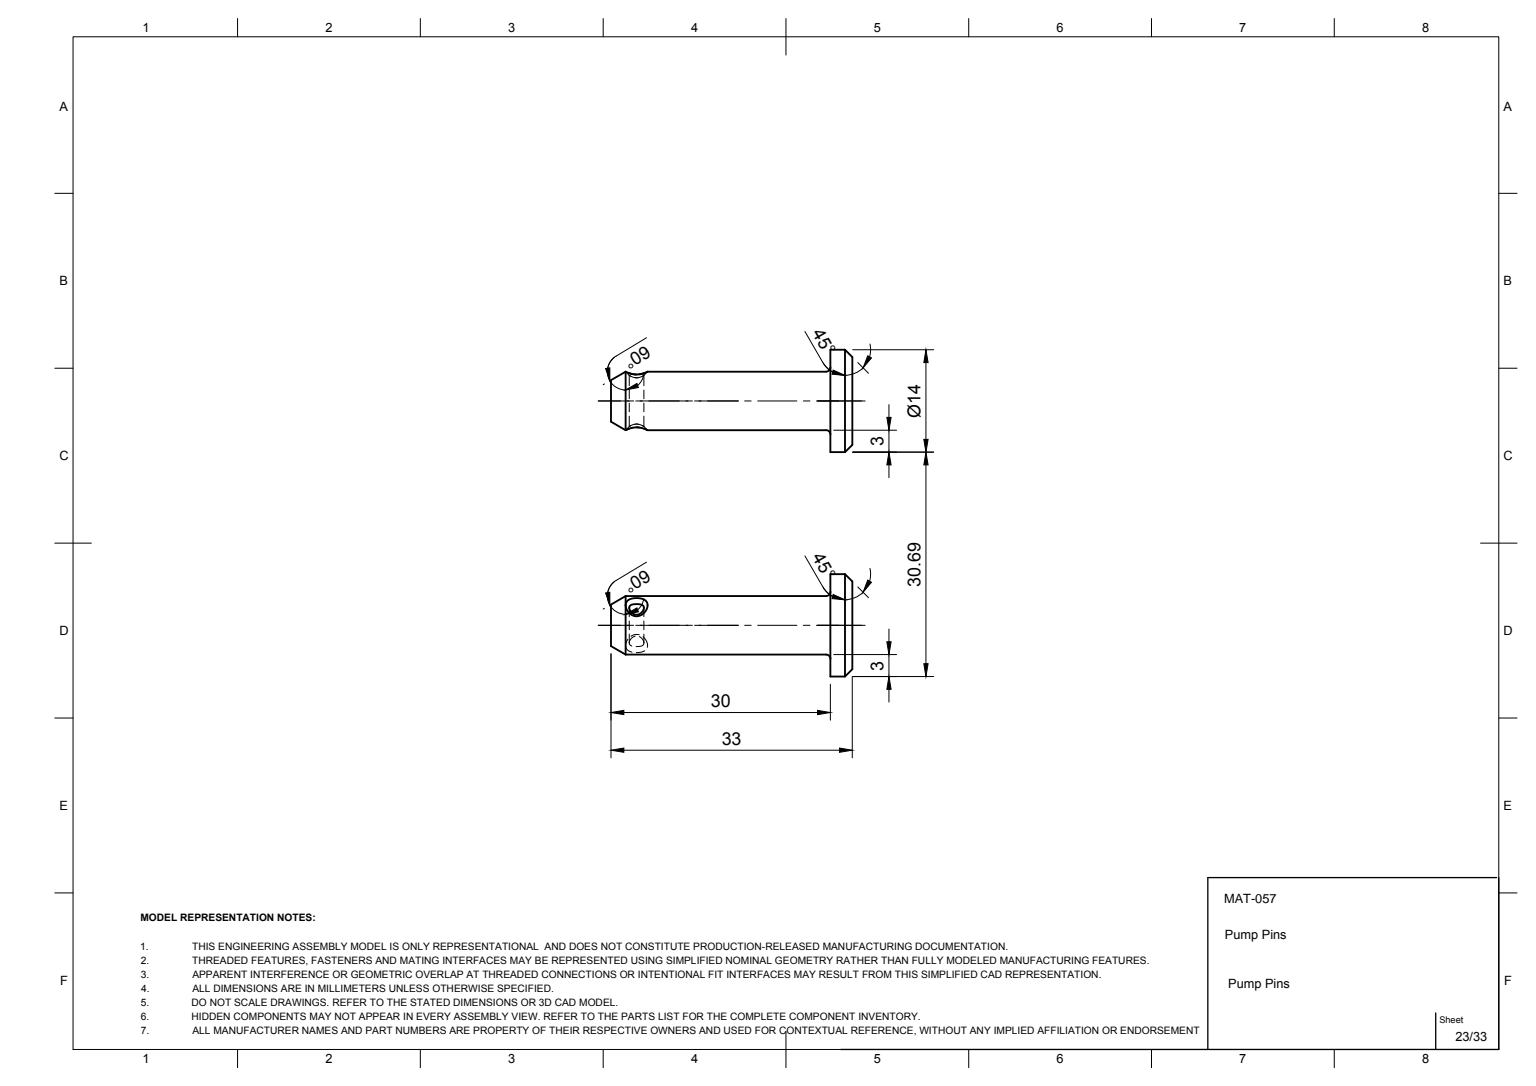
ISO-10303-21;
HEADER;
/* Generated by software containing ST-Developer
 * from STEP Tools, Inc. (www.steptools.com) 
 */

FILE_DESCRIPTION(
/* description */ ('STEP AP214', 'CAx-IF Rec.Pracs.---Representation and Presentation of Product Manufa
cturing Information (PMI)---4.0---2014-10-13'),
/* implementation_level */ '2;1');

FILE_NAME(
/* name */ 'Pump Pins.step',
/* time_stamp */ '2026-10-28T23:34:22+01:00',
/* author */ (''),
/* organization */ (''),
/* preprocessor_version */ 'ST-DEVELOPER v20.2',
/* originating_system */ 'Autodesk Translation Framework v15.17.0.0',
/* authorisation */ '');

FILE_SCHEMA (('AP242_MANAGED_MODEL_BASED_3D_ENGINEERING_MIM_LF { 1 0 10303 442 2 1 4 }'));
ENDSEC;

DATA;
#10=MECHANICAL_DESIGN_GEOMETRIC_PRESENTATION_REPRESENTATION('',(#264,#265),#27807);
#11=B_SPLINE_SURFACE_WITH_KNOTS('',1,3,((#21472,#21473,#21474,#21475,#21476,
#21477,#21478,#21479,#21480,#21481,#21482,#21483,#21484,#21485,#21486,#21487,
#21488,#21489),(#21490,#21491,#21492,#21493,#21494,#21495,#21496,#21497,
#21498,#21499,#21500,#21501,#21502,#21503,#21504,#21505,#21506,#21507)),
 .UNSPECIFIED.,.F.,.T.,.F.,(2,2),(4,2,2,2,2,2,2,2,4),(-5.33401314790998E-5,
1.0071581353373),(-0.00941606787651008,-0.00822939788115615,-0.00704272788580222,
-0.00585605789044829,-0.00466938789509436,-0.00348271789974043,-0.0022960479043865,
-0.00110937790903257,7.72920863213594E-5),.UNSPECIFIED.);
#12=B_SPLINE_SURFACE_WITH_KNOTS('',1,3,((#21574,#21575,#21576,#21577,#21578,
#21579,#21580,#21581,#21582,#21583,#21584,#21585,#21586,#21587,#21588,#21589,
#21590,#21591),(#21592,#21593,#21594,#21595,#21596,#21597,#21598,#21599,
#21600,#21601,#21602,#21603,#21604,#21605,#21606,#21607,#21608,#21609)),
 .UNSPECIFIED.,.F.,.T.,.F.,(2,2),(4,2,2,2,2,2,2,2,4),(-5.33401315292344E-5,
1.00729193620298),(-0.00941606787651008,-0.00822939788115615,-0.00704272788580222,
-0.00585605789044829,-0.00466938789509436,-0.00348271789974043,-0.0022960479043865,
-0.00110937790903257,7.72920863213577E-5),.UNSPECIFIED.);
#13=B_SPLINE_SURFACE_WITH_KNOTS('',1,3,((#21829,#21830,#21831,#21832,#21833,
#21834,#21835,#21836,#21837,#21838,#21839,#21840,#21841,#21842,#21843,#21844,
#21845,#21846),(#21847,#21848,#21849,#21850,#21851,#21852,#21853,#21854,
#21855,#21856,#21857,#21858,#21859,#21860,#21861,#21862,#21863,#21864)),
 .UNSPECIFIED.,.F.,.T.,.F.,(2,2),(4,2,2,2,2,2,2,2,4),(-4.93053323705934E-5,
1.01004399172031),(-0.00941606787651008,-0.00822939788115615,-0.00704272788580222,
-0.00585605789044829,-0.00466938789509436,-0.00348271789974043,-0.0022960479043865,
-0.00110937790903257,7.72920863213577E-5),.UNSPECIFIED.);
#14=B_SPLINE_SURFACE_WITH_KNOTS('',1,3,((#21865,#21866,#21867,#21868,#21869,
#21870,#21871,#21872,#21873,#21874,#21875,#21876,#21877,#21878,#21879,#21880,
#21881,#21882),(#21883,#21884,#21885,#21886,#21887,#21888,#21889,#21890,
#21891,#21892,#21893,#21894,#21895,#21896,#21897,#21898,#21899,#21900)),
 .UNSPECIFIED.,.F.,.T.,.F.,(2,2),(4,2,2,2,2,2,2,2,4),(-4.93053323625481E-5,
1.01010892051971),(-0.00941606787651008,-0.00822939788115615,-0.00704272788580222,
-0.00585605789044829,-0.00466938789509436,-0.00348271789974043,-0.0022960479043865,
-0.00110937790903257,7.72920863213594E-5),.UNSPECIFIED.);
#15=B_SPLINE_SURFACE_WITH_KNOTS('',1,3,((#21901,#21902,#21903,#21904,#21905,
#21906,#21907,#21908,#21909,#21910,#21911,#21912,#21913,#21914,#21915,#21916,
#21917,#21918),(#21919,#21920,#21921,#21922,#21923,#21924,#21925,#21926,
#21927,#21928,#21929,#21930,#21931,#21932,#21933,#21934,#21935,#21936)),
 .UNSPECIFIED.,.F.,.T.,.F.,(2,2),(4,2,2,2,2,2,2,2,4),(-4.62400267622051E-5,
1.00715813533735),(-0.00941606787651008,-0.00822939788115615,-0.00704272788580222,
-0.00585605789044829,-0.00466938789509436,-0.00348271789974043,-0.0022960479043865,
-0.00110937790903257,7.72920863213594E-5),.UNSPECIFIED.);
#16=B_SPLINE_SURFACE_WITH_KNOTS('',1,3,((#22003,#22004,#22005,#22006,#22007,
#22008,#22009,#22010,#22011,#22012,#22013,#22014,#22015,#22016,#22017,#22018,
#22019,#22020),(#22021,#22022,#22023,#22024,#22025,#22026,#22027,#22028,
#22029,#22030,#22031,#22032,#22033,#22034,#22035,#22036,#22037,#22038)),
 .UNSPECIFIED.,.F.,.T.,.F.,(2,2),(4,2,2,2,2,2,2,2,4),(-4.62400267636951E-5,
1.00729193620287),(-0.00941606787651008,-0.00822939788115615,-0.00704272788580222,
-0.00585605789044829,-0.00466938789509436,-0.00348271789974043,-0.0022960479043865,
-0.00110937790903257,7.72920863213577E-5),.UNSPECIFIED.);
#17=B_SPLINE_SURFACE_WITH_KNOTS('',1,3,((#22258,#22259,#22260,#22261,#22262,
#22263,#22264,#22265,#22266,#22267,#22268,#22269,#22270,#22271,#22272,#22273,
#22274,#22275),(#22276,#22277,#22278,#22279,#22280,#22281,#22282,#22283,
#22284,#22285,#22286,#22287,#22288,#22289,#22290,#22291,#22292,#22293)),
 .UNSPECIFIED.,.F.,.T.,.F.,(2,2),(4,2,2,2,2,2,2,2,4),(-4.93053323759633E-5,
1.00770004007163),(-0.00941606787651008,-0.00822939788115615,-0.00704272788580222,
-0.00585605789044829,-0.00466938789509436,-0.00348271789974043,-0.0022960479043865,
-0.00110937790903257,7.72920863213577E-5),.UNSPECIFIED.);
#18=B_SPLINE_SURFACE_WITH_KNOTS('',1,3,((#22294,#22295,#22296,#22297,#22298,
#22299,#22300,#22301,#22302,#22303,#22304,#22305,#22306,#22307,#22308,#22309,
#22310,#22311),(#22312,#22313,#22314,#22315,#22316,#22317,#22318,#22319,
#22320,#22321,#22322,#22323,#22324,#22325,#22326,#22327,#22328,#22329)),
 .UNSPECIFIED.,.F.,.T.,.F.,(2,2),(4,2,2,2,2,2,2,2,4),(-4.93053323767007E-5,
1.00811188664),(-0.00941606787651008,-0.00822939788115615,-0.00704272788580222,
-0.00585605789044829,-0.00466938789509436,-0.00348271789974043,-0.0022960479043865,
-0.00110937790903257,7.72920863213594E-5),.UNSPECIFIED.);
#218=SHAPE_REPRESENTATION_RELATIONSHIP('SRR','None',#27915,#240);
#240=ADVANCED_BREP_SHAPE_REPRESENTATION('',(#293,#294),#27795);
#264=STYLED_ITEM('',(#28063),#293);
#265=STYLED_ITEM('',(#28063),#294);
#293=MANIFOLD_SOLID_BREP('Body1',#12040);
#294=MANIFOLD_SOLID_BREP('Body2',#12041);
#414=FACE_BOUND('',#2492,.T.);
#415=FACE_BOUND('',#2506,.T.);
#665=PLANE('',#13280);
#666=PLANE('',#13281);
#667=PLANE('',#13282);
#668=PLANE('',#13299);
#669=PLANE('',#13300);
#670=PLANE('',#13301);
#832=TOROIDAL_SURFACE('',#13271,4.59999999999999,0.6);
#833=TOROIDAL_SURFACE('',#13290,4.59999999999999,0.6);
#904=B_SPLINE_CURVE_WITH_KNOTS('',3,(#21510,#21511,#21512,#21513,#21514,
#21515,#21516,#21517,#21518,#21519,#21520,#21521,#21522,#21523,#21524,#21525,
#21526,#21527,#21528,#21529,#21530,#21531,#21532,#21533,#21534,#21535,#21536,
#21537,#21538,#21539,#21540,#21541,#21542,#21543,#21544,#21545,#21546,#21547),
 .UNSPECIFIED.,.F.,.F.,(4,2,2,2,2,2,2,2,2,2,2,2,2,2,2,2,2,2,4),(1.00089634517109E-6,
0.0135124805886909,0.0270102893796787,0.0542554527433717,0.0725924484028551,
0.0831509031929542,0.0939203394783847,0.114150905777324,0.132564433691206,
0.163148633358063,0.193616759129243,0.211927287774423,0.23206669119174,
0.242799260198686,0.253302631405238,0.27156325585088,0.298722401714205,
0.312167688321445,0.325612440221502),.UNSPECIFIED.);
#905=B_SPLINE_CURVE_WITH_KNOTS('',3,(#21551,#21552,#21553,#21554,#21555,
#21556,#21557,#21558,#21559,#21560,#21561,#21562,#21563,#21564,#21565,#21566,
#21567,#21568,#21569,#21570,#21571,#21572),.UNSPECIFIED.,.F.,.F.,(4,2,2,
2,2,2,2,2,2,2,4),(0.,0.0625283246425461,0.0937924869638204,0.125056649285095,
0.187584973927639,0.250113298570183,0.312641623212727,0.343905785533998,
0.359537866694632,0.375169947855267,0.500226597140354),.UNSPECIFIED.);
#906=B_SPLINE_CURVE_WITH_KNOTS('',3,(#21612,#21613,#21614,#21615,#21616,
#21617,#21618,#21619,#21620,#21621,#21622,#21623,#21624,#21625,#21626,#21627,
#21628,#21629,#21630,#21631,#21632,#21633,#21634,#21635,#21636,#21637,#21638,
#21639,#21640,#21641,#21642,#21643,#21644,#21645,#21646,#21647,#21648,#21649),
 .UNSPECIFIED.,.F.,.F.,(4,2,2,2,2,2,2,2,2,2,2,2,2,2,2,2,2,2,4),(1.00089547843557E-6,
0.0135124805885893,0.0270102893791961,0.0542554527419749,0.072592448400889,
0.0831509031907464,0.0939203394761004,0.1141509057748,0.132564433688463,
0.163148633354892,0.193616759125631,0.211927287770558,0.232066691187639,
0.242799260194547,0.253302631400942,0.271563255846155,0.298722401708962,
0.312167688315685,0.325612440214992),.UNSPECIFIED.);
#907=B_SPLINE_CURVE_WITH_KNOTS('',3,(#21653,#21654,#21655,#21656,#21657,
#21658,#21659,#21660,#21661,#21662,#21663,#21664,#21665,#21666,#21667,#21668,
#21669,#21670,#21671,#21672,#21673,#21674),.UNSPECIFIED.,.F.,.F.,(4,2,2,
2,2,2,2,2,2,2,4),(0.,0.0625305420531017,0.0937958130796483,0.125061084106195,
0.187591626159283,0.250122168212371,0.31265271026546,0.343917981292008,
0.359550616805279,0.37518325231855,0.500244336424745),.UNSPECIFIED.);
#908=B_SPLINE_CURVE_WITH_KNOTS('',3,(#21677,#21678,#21679,#21680,#21681,
#21682,#21683,#21684,#21685,#21686,#21687,#21688,#21689,#21690,#21691,#21692,
#21693,#21694,#21695,#21696,#21697,#21698,#21699,#21700,#21701,#21702,#21703,
#21704,#21705,#21706,#21707,#21708,#21709,#21710,#21711,#21712,#21713,#21714),
 .UNSPECIFIED.,.F.,.F.,(4,2,2,2,2,2,2,2,2,2,2,2,2,2,2,2,2,2,4),(0.,0.0303468331885949,
0.0404805816100016,0.0838349998679533,0.0899468517242951,0.0960856059764287,
0.119205002215768,0.140283020185445,0.159234503235151,0.176557837747224,
0.209013384982688,0.227277173706207,0.247357834439419,0.25806173913776,
0.268531153677092,0.286711917123732,0.300273063907743,0.310385248581606,
0.340667271090375),.UNSPECIFIED.);
#909=B_SPLINE_CURVE_WITH_KNOTS('',3,(#21716,#21717,#21718,#21719,#21720,
#21721,#21722,#21723,#21724,#21725,#21726,#21727,#21728,#21729,#21730,#21731,
#21732,#21733,#21734,#21735,#21736,#21737,#21738,#21739,#21740,#21741,#21742,
#21743,#21744,#21745,#21746,#21747,#21748,#21749,#21750,#21751,#21752,#21753),
 .UNSPECIFIED.,.F.,.F.,(4,2,2,2,2,2,2,2,2,2,2,2,2,2,2,2,2,2,4),(0.,0.0303468331885437,
0.0404805816098057,0.0838349998664512,0.0899468517228076,0.096085605973945,
0.119205002207746,0.140283020172398,0.159234503217531,0.176557837725533,
0.209013384952252,0.227277173670161,0.247357834397049,0.258061739092016,
0.268531153628422,0.286711917069987,0.300273063850531,0.310385248521581,
0.340667271021422),.UNSPECIFIED.);
#910=B_SPLINE_CURVE_WITH_KNOTS('',3,(#21764,#21765,#21766,#21767,#21768,
#21769,#21770,#21771,#21772,#21773,#21774,#21775,#21776,#21777,#21778,#21779,
#21780,#21781,#21782,#21783,#21784,#21785),.UNSPECIFIED.,.F.,.F.,(4,2,2,
2,2,2,2,2,2,2,4),(0.500226597140354,0.562698272497809,0.593934110176538,
0.625169947855266,0.687641623212725,0.750113298570185,0.812584973927644,
0.843820811606377,0.859438730445742,0.875056649285107,1.),.UNSPECIFIED.);
#911=B_SPLINE_CURVE_WITH_KNOTS('',3,(#21786,#21787,#21788,#21789,#21790,
#21791,#21792,#21793,#21794,#21795,#21796,#21797,#21798,#21799,#21800,#21801,
#21802,#21803,#21804,#21805,#21806,#21807,#21808,#21809),.UNSPECIFIED.,
 .F.,.F.,(4,2,2,2,2,2,2,2,2,2,2,4),(0.500244336424745,0.56271379437167,
0.593948523345132,0.609565887831865,0.625183252318598,0.687652710265505,
0.750122168212412,0.812591626159318,0.843826355132767,0.859443719619489,
0.87506108410621,1.),.UNSPECIFIED.);
#912=B_SPLINE_CURVE_WITH_KNOTS('',3,(#21939,#21940,#21941,#21942,#21943,
#21944,#21945,#21946,#21947,#21948,#21949,#21950,#21951,#21952,#21953,#21954,
#21955,#21956,#21957,#21958,#21959,#21960,#21961,#21962,#21963,#21964,#21965,
#21966,#21967,#21968,#21969,#21970,#21971,#21972,#21973,#21974,#21975,#21976),
 .UNSPECIFIED.,.F.,.F.,(4,2,2,2,2,2,2,2,2,2,2,2,2,2,2,2,2,2,4),(1.00089633934029E-6,
0.0135124805888077,0.0270102893800241,0.0542554527437976,0.0725924484033422,
0.0831509031934888,0.0939203394789252,0.114150905777859,0.132564433691779,
0.163148633358663,0.193616759129903,0.211927287775115,0.232066691192426,
0.242799260199493,0.253302631405774,0.271563255850625,0.298722401712991,
0.312167688319558,0.32561244021873),.UNSPECIFIED.);
#913=B_SPLINE_CURVE_WITH_KNOTS('',3,(#21980,#21981,#21982,#21983,#21984,
#21985,#21986,#21987,#21988,#21989,#21990,#21991,#21992,#21993,#21994,#21995,
#21996,#21997,#21998,#21999,#22000,#22001),.UNSPECIFIED.,.F.,.F.,(4,2,2,
2,2,2,2,2,2,2,4),(0.,0.062528324642553,0.0937924869638229,0.125056649285093,
0.187584973927634,0.250113298570175,0.312641623212717,0.343905785533987,
0.359537866694625,0.375169947855263,0.500226597140362),.UNSPECIFIED.);
#914=B_SPLINE_CURVE_WITH_KNOTS('',3,(#22041,#22042,#22043,#22044,#22045,
#22046,#22047,#22048,#22049,#22050,#22051,#22052,#22053,#22054,#22055,#22056,
#22057,#22058,#22059,#22060,#22061,#22062,#22063,#22064,#22065,#22066,#22067,
#22068,#22069,#22070,#22071,#22072,#22073,#22074,#22075,#22076,#22077,#22078),
 .UNSPECIFIED.,.F.,.F.,(4,2,2,2,2,2,2,2,2,2,2,2,2,2,2,2,2,2,4),(1.00089547198642E-6,
0.0135124805886458,0.0270102893792894,0.0542554527414999,0.0725924484001046,
0.0831509031898948,0.0939203394752058,0.114150905773714,0.132564433687167,
0.163148633353336,0.193616759123885,0.211927287768641,0.232066691185389,
0.242799260192144,0.253302631398652,0.27156325584398,0.29872240170682,0.312167688313921,
0.32561244021362),.UNSPECIFIED.);
#915=B_SPLINE_CURVE_WITH_KNOTS('',3,(#22082,#22083,#22084,#22085,#22086,
#22087,#22088,#22089,#22090,#22091,#22092,#22093,#22094,#22095,#22096,#22097,
#22098,#22099,#22100,#22101,#22102,#22103),.UNSPECIFIED.,.F.,.F.,(4,2,2,
2,2,2,2,2,2,2,4),(0.,0.0625305420531068,0.0937958130796515,0.125061084106196,
0.187591626159282,0.250122168212368,0.312652710265454,0.343917981291998,
0.359550616805267,0.375183252318535,0.500244336424746),.UNSPECIFIED.);
#916=B_SPLINE_CURVE_WITH_KNOTS('',3,(#22106,#22107,#22108,#22109,#22110,
#22111,#22112,#22113,#22114,#22115,#22116,#22117,#22118,#22119,#22120,#22121,
#22122,#22123,#22124,#22125,#22126,#22127,#22128,#22129,#22130,#22131,#22132,
#22133,#22134,#22135,#22136,#22137,#22138,#22139,#22140,#22141,#22142,#22143),
 .UNSPECIFIED.,.F.,.F.,(4,2,2,2,2,2,2,2,2,2,2,2,2,2,2,2,2,2,4),(0.,0.0303468331886201,
0.0404805816100005,0.0838349998685196,0.0899468517249421,0.0960856059763945,
0.119205002212153,0.140283020178524,0.159234503225117,0.176557837734437,
0.209013384964693,0.227277173685149,0.247357834414858,0.25806173911128,
0.268531153648718,0.286711917091893,0.300273063873447,0.310385248545583,
0.340667271049151),.UNSPECIFIED.);
#917=B_SPLINE_CURVE_WITH_KNOTS('',3,(#22145,#22146,#22147,#22148,#22149,
#22150,#22151,#22152,#22153,#22154,#22155,#22156,#22157,#22158,#22159,#22160,
#22161,#22162,#22163,#22164,#22165,#22166,#22167,#22168,#22169,#22170,#22171,
#22172,#22173,#22174,#22175,#22176,#22177,#22178,#22179,#22180,#22181,#22182),
 .UNSPECIFIED.,.F.,.F.,(4,2,2,2,2,2,2,2,2,2,2,2,2,2,2,2,2,2,4),(0.,0.0303468331885424,
0.0404805816097377,0.0838349998665984,0.0899468517222195,0.0960856059733606,
0.119205002209305,0.140283020175775,0.159234503222523,0.176557837732021,
0.209013384962109,0.227277173682202,0.247357834411472,0.258061739107788,
0.268531153645427,0.28671191708922,0.300273063871285,0.310385248543308,
0.340667271045991),.UNSPECIFIED.);
#918=B_SPLINE_CURVE_WITH_KNOTS('',3,(#22193,#22194,#22195,#22196,#22197,
#22198,#22199,#22200,#22201,#22202,#22203,#22204,#22205,#22206,#22207,#22208,
#22209,#22210,#22211,#22212,#22213,#22214),.UNSPECIFIED.,.F.,.F.,(4,2,2,
2,2,2,2,2,2,2,4),(0.500226597140362,0.562698272497811,0.593934110176537,
0.625169947855262,0.687641623212722,0.750113298570183,0.812584973927644,
0.843820811606372,0.859438730445736,0.875056649285099,1.),.UNSPECIFIED.);
#919=B_SPLINE_CURVE_WITH_KNOTS('',3,(#22215,#22216,#22217,#22218,#22219,
#22220,#22221,#22222,#22223,#22224,#22225,#22226,#22227,#22228,#22229,#22230,
#22231,#22232,#22233,#22234,#22235,#22236,#22237,#22238),.UNSPECIFIED.,
 .F.,.F.,(4,2,2,2,2,2,2,2,2,2,2,4),(0.500244336424746,0.562713794371627,
0.593948523345067,0.609565887831793,0.625183252318519,0.687652710265425,
0.75012216821233,0.812591626159236,0.843826355132694,0.859443719619418,
0.875061084106143,1.),.UNSPECIFIED.);
#1151=CYLINDRICAL_SURFACE('',#13264,1.);
#1152=CYLINDRICAL_SURFACE('',#13269,4.);
#1153=CYLINDRICAL_SURFACE('',#13274,6.99999999999999);
#1154=CYLINDRICAL_SURFACE('',#13283,1.);
#1155=CYLINDRICAL_SURFACE('',#13288,4.00000000000001);
#1156=CYLINDRICAL_SURFACE('',#13293,7.);
#1706=FACE_OUTER_BOUND('',#2482,.T.);
#1707=FACE_OUTER_BOUND('',#2483,.T.);
#1708=FACE_OUTER_BOUND('',#2484,.T.);
#1709=FACE_OUTER_BOUND('',#2485,.T.);
#1710=FACE_OUTER_BOUND('',#2486,.T.);
#1711=FACE_OUTER_BOUND('',#2487,.T.);
#1712=FACE_OUTER_BOUND('',#2488,.T.);
#1713=FACE_OUTER_BOUND('',#2489,.T.);
#1714=FACE_OUTER_BOUND('',#2490,.T.);
#1715=FACE_OUTER_BOUND('',#2491,.T.);
#1716=FACE_OUTER_BOUND('',#2493,.T.);
#1717=FACE_OUTER_BOUND('',#2494,.T.);
#1718=FACE_OUTER_BOUND('',#2495,.T.);
#1719=FACE_OUTER_BOUND('',#2496,.T.);
#1720=FACE_OUTER_BOUND('',#2497,.T.);
#1721=FACE_OUTER_BOUND('',#2498,.T.);
#1722=FACE_OUTER_BOUND('',#2499,.T.);
#1723=FACE_OUTER_BOUND('',#2500,.T.);
#1724=FACE_OUTER_BOUND('',#2501,.T.);
#1725=FACE_OUTER_BOUND('',#2502,.T.);
#1726=FACE_OUTER_BOUND('',#2503,.T.);
#1727=FACE_OUTER_BOUND('',#2504,.T.);
#1728=FACE_OUTER_BOUND('',#2505,.T.);
#1729=FACE_OUTER_BOUND('',#2507,.T.);
#1730=FACE_OUTER_BOUND('',#2508,.T.);
#1731=FACE_OUTER_BOUND('',#2509,.T.);
#2482=EDGE_LOOP('',(#10163,#10164,#10165,#10166));
#2483=EDGE_LOOP('',(#10167,#10168,#10169,#10170));
#2484=EDGE_LOOP('',(#10171,#10172,#10173,#10174,#10175,#10176));
#2485=EDGE_LOOP('',(#10177,#10178,#10179,#10180,#10181));
#2486=EDGE_LOOP('',(#10182,#10183,#10184,#10185,#10186,#10187,#10188,#10189,
#10190));
#2487=EDGE_LOOP('',(#10191,#10192,#10193,#10194));
#2488=EDGE_LOOP('',(#10195,#10196,#10197,#10198,#10199));
#2489=EDGE_LOOP('',(#10200,#10201,#10202,#10203,#10204));
#2490=EDGE_LOOP('',(#10205));
#2491=EDGE_LOOP('',(#10206));
#2492=EDGE_LOOP('',(#10207));
#2493=EDGE_LOOP('',(#10208));
#2494=EDGE_LOOP('',(#10209,#10210,#10211,#10212));
#2495=EDGE_LOOP('',(#10213,#10214,#10215,#10216));
#2496=EDGE_LOOP('',(#10217,#10218,#10219,#10220));
#2497=EDGE_LOOP('',(#10221,#10222,#10223,#10224));
#2498=EDGE_LOOP('',(#10225,#10226,#10227,#10228,#10229,#10230));
#2499=EDGE_LOOP('',(#10231,#10232,#10233,#10234,#10235));
#2500=EDGE_LOOP('',(#10236,#10237,#10238,#10239,#10240,#10241,#10242,#10243,
#10244));
#2501=EDGE_LOOP('',(#10245,#10246,#10247,#10248));
#2502=EDGE_LOOP('',(#10249,#10250,#10251,#10252,#10253));
#2503=EDGE_LOOP('',(#10254,#10255,#10256,#10257,#10258));
#2504=EDGE_LOOP('',(#10259));
#2505=EDGE_LOOP('',(#10260));
#2506=EDGE_LOOP('',(#10261));
#2507=EDGE_LOOP('',(#10262));
#2508=EDGE_LOOP('',(#10263,#10264,#10265,#10266));
#2509=EDGE_LOOP('',(#10267,#10268,#10269,#10270));
#3344=LINE('',#21549,#4164);
#3345=LINE('',#21573,#4165);
#3346=LINE('',#21651,#4166);
#3347=LINE('',#21675,#4167);
#3348=LINE('',#21715,#4168);
#3349=LINE('',#21757,#4169);
#3350=LINE('',#21763,#4170);
#3351=LINE('',#21820,#4171);
#3352=LINE('',#21824,#4172);
#3353=LINE('',#21978,#4173);
#3354=LINE('',#22002,#4174);
#3355=LINE('',#22080,#4175);
#3356=LINE('',#22104,#4176);
#3357=LINE('',#22144,#4177);
#3358=LINE('',#22186,#4178);
#3359=LINE('',#22192,#4179);
#3360=LINE('',#22249,#4180);
#3361=LINE('',#22253,#4181);
#4164=VECTOR('',#16254,10.);
#4165=VECTOR('',#16255,10.);
#4166=VECTOR('',#16256,10.);
#4167=VECTOR('',#16257,10.);
#4168=VECTOR('',#16260,1.);
#4169=VECTOR('',#16265,4.);
#4170=VECTOR('',#16274,4.);
#4171=VECTOR('',#16287,6.99999999999999);
#4172=VECTOR('',#16292,5.99999999999997);
#4173=VECTOR('',#16301,10.);
#4174=VECTOR('',#16302,10.);
#4175=VECTOR('',#16303,10.);
#4176=VECTOR('',#16304,10.);
#4177=VECTOR('',#16307,1.);
#4178=VECTOR('',#16312,4.00000000000001);
#4179=VECTOR('',#16321,4.00000000000001);
#4180=VECTOR('',#16334,7.);
#4181=VECTOR('',#16339,5.99999999999998);
#4833=CIRCLE('',#13266,4.);
#4834=CIRCLE('',#13267,2.84529946162073);
#4835=CIRCLE('',#13268,4.);
#4836=CIRCLE('',#13270,4.);
#4837=CIRCLE('',#13272,4.59999999999999);
#4838=CIRCLE('',#13273,0.6);
#4839=CIRCLE('',#13275,6.99999999999999);
#4840=CIRCLE('',#13276,6.99999999999999);
#4841=CIRCLE('',#13277,6.99999999999999);
#4842=CIRCLE('',#13279,5.99999999999997);
#4843=CIRCLE('',#13285,4.00000000000001);
#4844=CIRCLE('',#13286,2.84529946162074);
#4845=CIRCLE('',#13287,4.00000000000001);
#4846=CIRCLE('',#13289,4.00000000000001);
#4847=CIRCLE('',#13291,4.6);
#4848=CIRCLE('',#13292,0.6);
#4849=CIRCLE('',#13294,7.);
#4850=CIRCLE('',#13295,7.);
#4851=CIRCLE('',#13296,7.);
#4852=CIRCLE('',#13298,5.99999999999998);
#5781=VERTEX_POINT('',#21508);
#5782=VERTEX_POINT('',#21509);
#5783=VERTEX_POINT('',#21548);
#5784=VERTEX_POINT('',#21550);
#5785=VERTEX_POINT('',#21610);
#5786=VERTEX_POINT('',#21611);
#5787=VERTEX_POINT('',#21650);
#5788=VERTEX_POINT('',#21652);
#5789=VERTEX_POINT('',#21756);
#5790=VERTEX_POINT('',#21761);
#5791=VERTEX_POINT('',#21811);
#5792=VERTEX_POINT('',#21815);
#5793=VERTEX_POINT('',#21816);
#5794=VERTEX_POINT('',#21819);
#5795=VERTEX_POINT('',#21823);
#5796=VERTEX_POINT('',#21937);
#5797=VERTEX_POINT('',#21938);
#5798=VERTEX_POINT('',#21977);
#5799=VERTEX_POINT('',#21979);
#5800=VERTEX_POINT('',#22039);
#5801=VERTEX_POINT('',#22040);
#5802=VERTEX_POINT('',#22079);
#5803=VERTEX_POINT('',#22081);
#5804=VERTEX_POINT('',#22185);
#5805=VERTEX_POINT('',#22190);
#5806=VERTEX_POINT('',#22240);
#5807=VERTEX_POINT('',#22244);
#5808=VERTEX_POINT('',#22245);
#5809=VERTEX_POINT('',#22248);
#5810=VERTEX_POINT('',#22252);
#7294=EDGE_CURVE('',#5781,#5782,#904,.T.);
#7295=EDGE_CURVE('',#5781,#5783,#3344,.T.);
#7296=EDGE_CURVE('',#5784,#5783,#905,.T.);
#7297=EDGE_CURVE('',#5782,#5784,#3345,.T.);
#7298=EDGE_CURVE('',#5785,#5786,#906,.T.);
#7299=EDGE_CURVE('',#5785,#5787,#3346,.T.);
#7300=EDGE_CURVE('',#5788,#5787,#907,.T.);
#7301=EDGE_CURVE('',#5786,#5788,#3347,.T.);
#7302=EDGE_CURVE('',#5782,#5781,#908,.T.);
#7303=EDGE_CURVE('',#5781,#5785,#3348,.T.);
#7304=EDGE_CURVE('',#5786,#5785,#909,.T.);
#7305=EDGE_CURVE('',#5784,#5788,#4833,.T.);
#7306=EDGE_CURVE('',#5784,#5789,#3349,.T.);
#7307=EDGE_CURVE('',#5789,#5789,#4834,.T.);
#7308=EDGE_CURVE('',#5788,#5784,#4835,.T.);
#7309=EDGE_CURVE('',#5790,#5790,#4836,.T.);
#7310=EDGE_CURVE('',#5790,#5783,#3350,.T.);
#7311=EDGE_CURVE('',#5783,#5784,#910,.T.);
#7312=EDGE_CURVE('',#5787,#5788,#911,.T.);
#7313=EDGE_CURVE('',#5791,#5791,#4837,.T.);
#7314=EDGE_CURVE('',#5791,#5790,#4838,.T.);
#7315=EDGE_CURVE('',#5792,#5793,#4839,.T.);
#7316=EDGE_CURVE('',#5793,#5792,#4840,.T.);
#7317=EDGE_CURVE('',#5793,#5794,#3351,.T.);
#7318=EDGE_CURVE('',#5794,#5794,#4841,.T.);
#7319=EDGE_CURVE('',#5792,#5795,#3352,.T.);
#7320=EDGE_CURVE('',#5795,#5795,#4842,.T.);
#7321=EDGE_CURVE('',#5796,#5797,#912,.T.);
#7322=EDGE_CURVE('',#5796,#5798,#3353,.T.);
#7323=EDGE_CURVE('',#5799,#5798,#913,.T.);
#7324=EDGE_CURVE('',#5797,#5799,#3354,.T.);
#7325=EDGE_CURVE('',#5800,#5801,#914,.T.);
#7326=EDGE_CURVE('',#5800,#5802,#3355,.T.);
#7327=EDGE_CURVE('',#5803,#5802,#915,.T.);
#7328=EDGE_CURVE('',#5801,#5803,#3356,.T.);
#7329=EDGE_CURVE('',#5797,#5796,#916,.T.);
#7330=EDGE_CURVE('',#5796,#5800,#3357,.T.);
#7331=EDGE_CURVE('',#5801,#5800,#917,.T.);
#7332=EDGE_CURVE('',#5799,#5803,#4843,.T.);
#7333=EDGE_CURVE('',#5799,#5804,#3358,.T.);
#7334=EDGE_CURVE('',#5804,#5804,#4844,.T.);
#7335=EDGE_CURVE('',#5803,#5799,#4845,.T.);
#7336=EDGE_CURVE('',#5805,#5805,#4846,.T.);
#7337=EDGE_CURVE('',#5805,#5798,#3359,.T.);
#7338=EDGE_CURVE('',#5798,#5799,#918,.T.);
#7339=EDGE_CURVE('',#5802,#5803,#919,.T.);
#7340=EDGE_CURVE('',#5806,#5806,#4847,.T.);
#7341=EDGE_CURVE('',#5806,#5805,#4848,.T.);
#7342=EDGE_CURVE('',#5807,#5808,#4849,.T.);
#7343=EDGE_CURVE('',#5808,#5807,#4850,.T.);
#7344=EDGE_CURVE('',#5808,#5809,#3360,.T.);
#7345=EDGE_CURVE('',#5809,#5809,#4851,.T.);
#7346=EDGE_CURVE('',#5807,#5810,#3361,.T.);
#7347=EDGE_CURVE('',#5810,#5810,#4852,.T.);
#10163=ORIENTED_EDGE('',*,*,#7294,.F.);
#10164=ORIENTED_EDGE('',*,*,#7295,.T.);
#10165=ORIENTED_EDGE('',*,*,#7296,.F.);
#10166=ORIENTED_EDGE('',*,*,#7297,.F.);
#10167=ORIENTED_EDGE('',*,*,#7298,.F.);
#10168=ORIENTED_EDGE('',*,*,#7299,.T.);
#10169=ORIENTED_EDGE('',*,*,#7300,.F.);
#10170=ORIENTED_EDGE('',*,*,#7301,.F.);
#10171=ORIENTED_EDGE('',*,*,#7302,.T.);
#10172=ORIENTED_EDGE('',*,*,#7303,.T.);
#10173=ORIENTED_EDGE('',*,*,#7298,.T.);
#10174=ORIENTED_EDGE('',*,*,#7304,.T.);
#10175=ORIENTED_EDGE('',*,*,#7303,.F.);
#10176=ORIENTED_EDGE('',*,*,#7294,.T.);
#10177=ORIENTED_EDGE('',*,*,#7305,.F.);
#10178=ORIENTED_EDGE('',*,*,#7306,.T.);
#10179=ORIENTED_EDGE('',*,*,#7307,.T.);
#10180=ORIENTED_EDGE('',*,*,#7306,.F.);
#10181=ORIENTED_EDGE('',*,*,#7308,.F.);
#10182=ORIENTED_EDGE('',*,*,#7309,.F.);
#10183=ORIENTED_EDGE('',*,*,#7310,.T.);
#10184=ORIENTED_EDGE('',*,*,#7311,.T.);
#10185=ORIENTED_EDGE('',*,*,#7305,.T.);
#10186=ORIENTED_EDGE('',*,*,#7300,.T.);
#10187=ORIENTED_EDGE('',*,*,#7312,.T.);
#10188=ORIENTED_EDGE('',*,*,#7308,.T.);
#10189=ORIENTED_EDGE('',*,*,#7296,.T.);
#10190=ORIENTED_EDGE('',*,*,#7310,.F.);
#10191=ORIENTED_EDGE('',*,*,#7313,.F.);
#10192=ORIENTED_EDGE('',*,*,#7314,.T.);
#10193=ORIENTED_EDGE('',*,*,#7309,.T.);
#10194=ORIENTED_EDGE('',*,*,#7314,.F.);
#10195=ORIENTED_EDGE('',*,*,#7315,.F.);
#10196=ORIENTED_EDGE('',*,*,#7316,.F.);
#10197=ORIENTED_EDGE('',*,*,#7317,.T.);
#10198=ORIENTED_EDGE('',*,*,#7318,.T.);
#10199=ORIENTED_EDGE('',*,*,#7317,.F.);
#10200=ORIENTED_EDGE('',*,*,#7315,.T.);
#10201=ORIENTED_EDGE('',*,*,#7316,.T.);
#10202=ORIENTED_EDGE('',*,*,#7319,.T.);
#10203=ORIENTED_EDGE('',*,*,#7320,.F.);
#10204=ORIENTED_EDGE('',*,*,#7319,.F.);
#10205=ORIENTED_EDGE('',*,*,#7320,.T.);
#10206=ORIENTED_EDGE('',*,*,#7318,.F.);
#10207=ORIENTED_EDGE('',*,*,#7313,.T.);
#10208=ORIENTED_EDGE('',*,*,#7307,.F.);
#10209=ORIENTED_EDGE('',*,*,#7299,.F.);
#10210=ORIENTED_EDGE('',*,*,#7304,.F.);
#10211=ORIENTED_EDGE('',*,*,#7301,.T.);
#10212=ORIENTED_EDGE('',*,*,#7312,.F.);
#10213=ORIENTED_EDGE('',*,*,#7295,.F.);
#10214=ORIENTED_EDGE('',*,*,#7302,.F.);
#10215=ORIENTED_EDGE('',*,*,#7297,.T.);
#10216=ORIENTED_EDGE('',*,*,#7311,.F.);
#10217=ORIENTED_EDGE('',*,*,#7321,.F.);
#10218=ORIENTED_EDGE('',*,*,#7322,.T.);
#10219=ORIENTED_EDGE('',*,*,#7323,.F.);
#10220=ORIENTED_EDGE('',*,*,#7324,.F.);
#10221=ORIENTED_EDGE('',*,*,#7325,.F.);
#10222=ORIENTED_EDGE('',*,*,#7326,.T.);
#10223=ORIENTED_EDGE('',*,*,#7327,.F.);
#10224=ORIENTED_EDGE('',*,*,#7328,.F.);
#10225=ORIENTED_EDGE('',*,*,#7329,.T.);
#10226=ORIENTED_EDGE('',*,*,#7330,.T.);
#10227=ORIENTED_EDGE('',*,*,#7325,.T.);
#10228=ORIENTED_EDGE('',*,*,#7331,.T.);
#10229=ORIENTED_EDGE('',*,*,#7330,.F.);
#10230=ORIENTED_EDGE('',*,*,#7321,.T.);
#10231=ORIENTED_EDGE('',*,*,#7332,.F.);
#10232=ORIENTED_EDGE('',*,*,#7333,.T.);
#10233=ORIENTED_EDGE('',*,*,#7334,.T.);
#10234=ORIENTED_EDGE('',*,*,#7333,.F.);
#10235=ORIENTED_EDGE('',*,*,#7335,.F.);
#10236=ORIENTED_EDGE('',*,*,#7336,.F.);
#10237=ORIENTED_EDGE('',*,*,#7337,.T.);
#10238=ORIENTED_EDGE('',*,*,#7338,.T.);
#10239=ORIENTED_EDGE('',*,*,#7332,.T.);
#10240=ORIENTED_EDGE('',*,*,#7327,.T.);
#10241=ORIENTED_EDGE('',*,*,#7339,.T.);
#10242=ORIENTED_EDGE('',*,*,#7335,.T.);
#10243=ORIENTED_EDGE('',*,*,#7323,.T.);
#10244=ORIENTED_EDGE('',*,*,#7337,.F.);
#10245=ORIENTED_EDGE('',*,*,#7340,.F.);
#10246=ORIENTED_EDGE('',*,*,#7341,.T.);
#10247=ORIENTED_EDGE('',*,*,#7336,.T.);
#10248=ORIENTED_EDGE('',*,*,#7341,.F.);
#10249=ORIENTED_EDGE('',*,*,#7342,.F.);
#10250=ORIENTED_EDGE('',*,*,#7343,.F.);
#10251=ORIENTED_EDGE('',*,*,#7344,.T.);
#10252=ORIENTED_EDGE('',*,*,#7345,.T.);
#10253=ORIENTED_EDGE('',*,*,#7344,.F.);
#10254=ORIENTED_EDGE('',*,*,#7342,.T.);
#10255=ORIENTED_EDGE('',*,*,#7343,.T.);
#10256=ORIENTED_EDGE('',*,*,#7346,.T.);
#10257=ORIENTED_EDGE('',*,*,#7347,.F.);
#10258=ORIENTED_EDGE('',*,*,#7346,.F.);
#10259=ORIENTED_EDGE('',*,*,#7347,.T.);
#10260=ORIENTED_EDGE('',*,*,#7345,.F.);
#10261=ORIENTED_EDGE('',*,*,#7340,.T.);
#10262=ORIENTED_EDGE('',*,*,#7334,.F.);
#10263=ORIENTED_EDGE('',*,*,#7326,.F.);
#10264=ORIENTED_EDGE('',*,*,#7331,.F.);
#10265=ORIENTED_EDGE('',*,*,#7328,.T.);
#10266=ORIENTED_EDGE('',*,*,#7339,.F.);
#10267=ORIENTED_EDGE('',*,*,#7322,.F.);
#10268=ORIENTED_EDGE('',*,*,#7329,.F.);
#10269=ORIENTED_EDGE('',*,*,#7324,.T.);
#10270=ORIENTED_EDGE('',*,*,#7338,.F.);
#11308=CONICAL_SURFACE('',#13265,4.,0.5235987755983);
#11309=CONICAL_SURFACE('',#13278,5.99999999999997,0.78539816339745);
#11310=CONICAL_SURFACE('',#13284,4.00000000000001,0.5235987755983);
#11311=CONICAL_SURFACE('',#13297,5.99999999999998,0.78539816339745);
#11788=ADVANCED_FACE('',(#1706),#11,.T.);
#11789=ADVANCED_FACE('',(#1707),#12,.T.);
#11790=ADVANCED_FACE('',(#1708),#1151,.F.);
#11791=ADVANCED_FACE('',(#1709),#11308,.T.);
#11792=ADVANCED_FACE('',(#1710),#1152,.T.);
#11793=ADVANCED_FACE('',(#1711),#832,.F.);
#11794=ADVANCED_FACE('',(#1712),#1153,.T.);
#11795=ADVANCED_FACE('',(#1713),#11309,.T.);
#11796=ADVANCED_FACE('',(#1714),#665,.T.);
#11797=ADVANCED_FACE('',(#1715,#414),#666,.T.);
#11798=ADVANCED_FACE('',(#1716),#667,.T.);
#11799=ADVANCED_FACE('',(#1717),#13,.T.);
#11800=ADVANCED_FACE('',(#1718),#14,.T.);
#11801=ADVANCED_FACE('',(#1719),#15,.T.);
#11802=ADVANCED_FACE('',(#1720),#16,.T.);
#11803=ADVANCED_FACE('',(#1721),#1154,.F.);
#11804=ADVANCED_FACE('',(#1722),#11310,.T.);
#11805=ADVANCED_FACE('',(#1723),#1155,.T.);
#11806=ADVANCED_FACE('',(#1724),#833,.F.);
#11807=ADVANCED_FACE('',(#1725),#1156,.T.);
#11808=ADVANCED_FACE('',(#1726),#11311,.T.);
#11809=ADVANCED_FACE('',(#1727),#668,.T.);
#11810=ADVANCED_FACE('',(#1728,#415),#669,.T.);
#11811=ADVANCED_FACE('',(#1729),#670,.T.);
#11812=ADVANCED_FACE('',(#1730),#17,.T.);
#11813=ADVANCED_FACE('',(#1731),#18,.T.);
#12040=CLOSED_SHELL('',(#11788,#11789,#11790,#11791,#11792,#11793,#11794,
#11795,#11796,#11797,#11798,#11799,#11800));
#12041=CLOSED_SHELL('',(#11801,#11802,#11803,#11804,#11805,#11806,#11807,
#11808,#11809,#11810,#11811,#11812,#11813));
#13263=AXIS2_PLACEMENT_3D('',#21471,#16252,#16253);
#13264=AXIS2_PLACEMENT_3D('',#21676,#16258,#16259);
#13265=AXIS2_PLACEMENT_3D('',#21754,#16261,#16262);
#13266=AXIS2_PLACEMENT_3D('',#21755,#16263,#16264);
#13267=AXIS2_PLACEMENT_3D('',#21758,#16266,#16267);
#13268=AXIS2_PLACEMENT_3D('',#21759,#16268,#16269);
#13269=AXIS2_PLACEMENT_3D('',#21760,#16270,#16271);
#13270=AXIS2_PLACEMENT_3D('',#21762,#16272,#16273);
#13271=AXIS2_PLACEMENT_3D('',#21810,#16275,#16276);
#13272=AXIS2_PLACEMENT_3D('',#21812,#16277,#16278);
#13273=AXIS2_PLACEMENT_3D('',#21813,#16279,#16280);
#13274=AXIS2_PLACEMENT_3D('',#21814,#16281,#16282);
#13275=AXIS2_PLACEMENT_3D('',#21817,#16283,#16284);
#13276=AXIS2_PLACEMENT_3D('',#21818,#16285,#16286);
#13277=AXIS2_PLACEMENT_3D('',#21821,#16288,#16289);
#13278=AXIS2_PLACEMENT_3D('',#21822,#16290,#16291);
#13279=AXIS2_PLACEMENT_3D('',#21825,#16293,#16294);
#13280=AXIS2_PLACEMENT_3D('',#21826,#16295,#16296);
#13281=AXIS2_PLACEMENT_3D('',#21827,#16297,#16298);
#13282=AXIS2_PLACEMENT_3D('',#21828,#16299,#16300);
#13283=AXIS2_PLACEMENT_3D('',#22105,#16305,#16306);
#13284=AXIS2_PLACEMENT_3D('',#22183,#16308,#16309);
#13285=AXIS2_PLACEMENT_3D('',#22184,#16310,#16311);
#13286=AXIS2_PLACEMENT_3D('',#22187,#16313,#16314);
#13287=AXIS2_PLACEMENT_3D('',#22188,#16315,#16316);
#13288=AXIS2_PLACEMENT_3D('',#22189,#16317,#16318);
#13289=AXIS2_PLACEMENT_3D('',#22191,#16319,#16320);
#13290=AXIS2_PLACEMENT_3D('',#22239,#16322,#16323);
#13291=AXIS2_PLACEMENT_3D('',#22241,#16324,#16325);
#13292=AXIS2_PLACEMENT_3D('',#22242,#16326,#16327);
#13293=AXIS2_PLACEMENT_3D('',#22243,#16328,#16329);
#13294=AXIS2_PLACEMENT_3D('',#22246,#16330,#16331);
#13295=AXIS2_PLACEMENT_3D('',#22247,#16332,#16333);
#13296=AXIS2_PLACEMENT_3D('',#22250,#16335,#16336);
#13297=AXIS2_PLACEMENT_3D('',#22251,#16337,#16338);
#13298=AXIS2_PLACEMENT_3D('',#22254,#16340,#16341);
#13299=AXIS2_PLACEMENT_3D('',#22255,#16342,#16343);
#13300=AXIS2_PLACEMENT_3D('',#22256,#16344,#16345);
#13301=AXIS2_PLACEMENT_3D('',#22257,#16346,#16347);
#16252=DIRECTION('axis',(0.,0.,1.));
#16253=DIRECTION('refdir',(1.,0.,0.));
#16254=DIRECTION('',(0.487956526058392,0.511760784630642,0.707106306004447));
#16255=DIRECTION('',(0.487956174314074,0.51176044158493,-0.707106797009879));
#16256=DIRECTION('',(-0.487954254662986,-0.511762949542871,0.70710630659857));
#16257=DIRECTION('',(-0.487956174313991,-0.511760441584974,-0.707106797009905));
#16258=DIRECTION('center_axis',(-0.690074255005153,-0.72373857336685,7.51590717679369E-17));
#16259=DIRECTION('ref_axis',(-5.18653404571379E-17,-5.43955193769033E-17,
-1.));
#16260=DIRECTION('',(-0.690074255005153,-0.72373857336685,7.51590717679369E-17));
#16261=DIRECTION('center_axis',(8.42524722855705E-17,2.35148579188733E-17,
1.));
#16262=DIRECTION('ref_axis',(-0.690074255005155,-0.723738573366849,7.5159071767937E-17));
#16263=DIRECTION('center_axis',(8.42524722855705E-17,2.35148579188733E-17,
1.));
#16264=DIRECTION('ref_axis',(-0.690074255005155,-0.723738573366849,7.5159071767937E-17));
#16265=DIRECTION('',(-0.345037127502578,-0.361869286683425,-0.866025403784438));
#16266=DIRECTION('center_axis',(8.42524722855705E-17,2.35148579188733E-17,
1.));
#16267=DIRECTION('ref_axis',(-0.690074255005155,-0.723738573366848,7.5159071767937E-17));
#16268=DIRECTION('center_axis',(8.42524722855705E-17,2.35148579188733E-17,
1.));
#16269=DIRECTION('ref_axis',(-0.690074255005155,-0.723738573366849,7.5159071767937E-17));
#16270=DIRECTION('center_axis',(8.42524722855705E-17,2.35148579188733E-17,
1.));
#16271=DIRECTION('ref_axis',(-0.690074255005155,-0.723738573366849,7.5159071767937E-17));
#16272=DIRECTION('center_axis',(8.42524722855705E-17,2.35148579188733E-17,
1.));
#16273=DIRECTION('ref_axis',(-0.690074255005155,-0.723738573366849,7.5159071767937E-17));
#16274=DIRECTION('',(-8.42524722855704E-17,-2.35148579188733E-17,-1.));
#16275=DIRECTION('center_axis',(8.42524722855705E-17,2.35148579188733E-17,
1.));
#16276=DIRECTION('ref_axis',(-0.690074255005153,-0.723738573366849,0.));
#16277=DIRECTION('center_axis',(8.42524722855705E-17,2.35148579188733E-17,
1.));
#16278=DIRECTION('ref_axis',(-0.690074255005155,-0.723738573366848,7.5159071767937E-17));
#16279=DIRECTION('center_axis',(0.723738573366851,-0.690074255005152,-4.47497660346704E-17));
#16280=DIRECTION('ref_axis',(0.690074255005152,0.723738573366851,0.));
#16281=DIRECTION('center_axis',(8.42524722855705E-17,2.35148579188733E-17,
1.));
#16282=DIRECTION('ref_axis',(-0.690074255005154,-0.723738573366849,7.51590717679369E-17));
#16283=DIRECTION('center_axis',(8.42524722855705E-17,2.35148579188733E-17,
1.));
#16284=DIRECTION('ref_axis',(-0.690074255005154,-0.723738573366849,7.51590717679369E-17));
#16285=DIRECTION('center_axis',(8.42524722855705E-17,2.35148579188733E-17,
1.));
#16286=DIRECTION('ref_axis',(-0.690074255005154,-0.723738573366849,7.51590717679369E-17));
#16287=DIRECTION('',(-8.42524722855705E-17,-2.35148579188733E-17,-1.));
#16288=DIRECTION('center_axis',(8.42524722855705E-17,2.35148579188733E-17,
1.));
#16289=DIRECTION('ref_axis',(-0.690074255005154,-0.723738573366849,7.51590717679369E-17));
#16290=DIRECTION('center_axis',(-8.42524722855705E-17,-2.35148579188733E-17,
-1.));
#16291=DIRECTION('ref_axis',(0.690074255005153,0.72373857336685,-7.51590717679369E-17));
#16292=DIRECTION('',(0.487956185236399,0.511760453033977,0.707106781186547));
#16293=DIRECTION('center_axis',(8.42524722855705E-17,2.35148579188733E-17,
1.));
#16294=DIRECTION('ref_axis',(-0.690074255005153,-0.72373857336685,7.51590717679369E-17));
#16295=DIRECTION('center_axis',(8.42524722855704E-17,2.35148579188733E-17,
1.));
#16296=DIRECTION('ref_axis',(-0.690074255005153,-0.72373857336685,7.51590717679369E-17));
#16297=DIRECTION('center_axis',(-8.42524722855704E-17,-2.35148579188733E-17,
-1.));
#16298=DIRECTION('ref_axis',(0.690074255005153,0.72373857336685,-7.51590717679369E-17));
#16299=DIRECTION('center_axis',(-8.42524722855704E-17,-2.35148579188733E-17,
-1.));
#16300=DIRECTION('ref_axis',(0.690074255005153,0.72373857336685,-7.51590717679369E-17));
#16301=DIRECTION('',(0.0359217337292158,-0.706194237483284,0.707106306004472));
#16302=DIRECTION('',(0.0359217266067779,-0.706193746205675,-0.707106797009888));
#16303=DIRECTION('',(-0.0359248674940963,0.706194077477286,0.707106306598617));
#16304=DIRECTION('',(-0.0359217266067779,0.706193746205675,-0.707106797009888));
#16305=DIRECTION('center_axis',(-0.0508009940819139,0.998708795896126,-1.92022413686896E-17));
#16306=DIRECTION('ref_axis',(9.7549295013028E-19,-1.91774473558307E-17,
-1.));
#16307=DIRECTION('',(-0.0508009940819138,0.998708795896126,-1.92022413686896E-17));
#16308=DIRECTION('center_axis',(8.42672643859301E-17,2.35134628477836E-17,
1.));
#16309=DIRECTION('ref_axis',(-0.0508009940819175,0.998708795896126,-1.92022413686893E-17));
#16310=DIRECTION('center_axis',(8.42672643859301E-17,2.35134628477836E-17,
1.));
#16311=DIRECTION('ref_axis',(-0.0508009940819175,0.998708795896126,-1.92022413686893E-17));
#16312=DIRECTION('',(-0.0254004970409589,0.499354397948064,-0.866025403784438));
#16313=DIRECTION('center_axis',(8.42672643859301E-17,2.35134628477836E-17,
1.));
#16314=DIRECTION('ref_axis',(-0.0508009940819193,0.998708795896126,-1.92022413686891E-17));
#16315=DIRECTION('center_axis',(8.42672643859301E-17,2.35134628477836E-17,
1.));
#16316=DIRECTION('ref_axis',(-0.0508009940819175,0.998708795896126,-1.92022413686893E-17));
#16317=DIRECTION('center_axis',(8.42672643859301E-17,2.35134628477836E-17,
1.));
#16318=DIRECTION('ref_axis',(-0.0508009940819175,0.998708795896126,-1.92022413686893E-17));
#16319=DIRECTION('center_axis',(8.42672643859301E-17,2.35134628477836E-17,
1.));
#16320=DIRECTION('ref_axis',(-0.0508009940819175,0.998708795896126,-1.92022413686893E-17));
#16321=DIRECTION('',(-8.42672643859301E-17,-2.35134628477836E-17,-1.));
#16322=DIRECTION('center_axis',(8.42672643859301E-17,2.35134628477836E-17,
1.));
#16323=DIRECTION('ref_axis',(-0.0508009940819075,0.998708795896126,0.));
#16324=DIRECTION('center_axis',(8.42672643859301E-17,2.35134628477836E-17,
1.));
#16325=DIRECTION('ref_axis',(-0.0508009940819092,0.998708795896126,-1.920224136869E-17));
#16326=DIRECTION('center_axis',(-0.998708795896126,-0.0508009940819131,
8.53529654353083E-17));
#16327=DIRECTION('ref_axis',(0.0508009940819131,-0.998708795896126,0.));
#16328=DIRECTION('center_axis',(8.42672643859301E-17,2.35134628477836E-17,
1.));
#16329=DIRECTION('ref_axis',(-0.0508009940819137,0.998708795896126,-1.92022413686896E-17));
#16330=DIRECTION('center_axis',(8.42672643859301E-17,2.35134628477836E-17,
1.));
#16331=DIRECTION('ref_axis',(-0.0508009940819137,0.998708795896126,-1.92022413686896E-17));
#16332=DIRECTION('center_axis',(8.42672643859301E-17,2.35134628477836E-17,
1.));
#16333=DIRECTION('ref_axis',(-0.0508009940819137,0.998708795896126,-1.92022413686896E-17));
#16334=DIRECTION('',(-8.42672643859301E-17,-2.35134628477836E-17,-1.));
#16335=DIRECTION('center_axis',(8.42672643859301E-17,2.35134628477836E-17,
1.));
#16336=DIRECTION('ref_axis',(-0.0508009940819137,0.998708795896126,-1.92022413686896E-17));
#16337=DIRECTION('center_axis',(-8.42672643859301E-17,-2.35134628477836E-17,
-1.));
#16338=DIRECTION('ref_axis',(0.0508009940819178,-0.998708795896126,1.92022413686892E-17));
#16339=DIRECTION('',(0.0359217274063417,-0.706193762008803,0.707106781186547));
#16340=DIRECTION('center_axis',(8.42672643859301E-17,2.35134628477836E-17,
1.));
#16341=DIRECTION('ref_axis',(-0.0508009940819178,0.998708795896126,-1.92022413686892E-17));
#16342=DIRECTION('center_axis',(8.42672643859301E-17,2.35134628477836E-17,
1.));
#16343=DIRECTION('ref_axis',(-0.0508009940819138,0.998708795896126,-1.92022413686896E-17));
#16344=DIRECTION('center_axis',(-8.42672643859301E-17,-2.35134628477836E-17,
-1.));
#16345=DIRECTION('ref_axis',(0.0508009940819138,-0.998708795896126,1.92022413686896E-17));
#16346=DIRECTION('center_axis',(-8.42672643859301E-17,-2.35134628477836E-17,
-1.));
#16347=DIRECTION('ref_axis',(0.0508009940819138,-0.998708795896126,1.92022413686896E-17));
#21471=CARTESIAN_POINT('',(0.,0.,0.));
#21472=CARTESIAN_POINT('Ctrl Pts',(241.704224565777,155.65704992868,244.573619803768));
#21473=CARTESIAN_POINT('Ctrl Pts',(241.510068395548,155.841112484094,244.574122853875));
#21474=CARTESIAN_POINT('Ctrl Pts',(241.271802936649,155.964045706855,244.684411798912));
#21475=CARTESIAN_POINT('Ctrl Pts',(240.885055878546,156.088013810182,245.049510693237));
#21476=CARTESIAN_POINT('Ctrl Pts',(240.747008314468,156.102746965415,245.307955179719));
#21477=CARTESIAN_POINT('Ctrl Pts',(240.747915979192,156.102607114311,245.84060223374));
#21478=CARTESIAN_POINT('Ctrl Pts',(240.88541559932,156.087955834116,246.097804076277));
#21479=CARTESIAN_POINT('Ctrl Pts',(241.272276604401,155.963830882667,246.463437960953));
#21480=CARTESIAN_POINT('Ctrl Pts',(241.511138824461,155.840473431548,246.573503411772));
#21481=CARTESIAN_POINT('Ctrl Pts',(241.899470444745,155.471564785668,246.573627286256));
#21482=CARTESIAN_POINT('Ctrl Pts',(242.031853219533,155.239145808301,246.462784974605));
#21483=CARTESIAN_POINT('Ctrl Pts',(242.173429602105,154.859535412975,246.097307277076));
#21484=CARTESIAN_POINT('Ctrl Pts',(242.194992380974,154.72208775409,245.8387163343));
#21485=CARTESIAN_POINT('Ctrl Pts',(242.19477499151,154.723076345322,245.306032501962));
#21486=CARTESIAN_POINT('Ctrl Pts',(242.173220430076,154.860146597241,245.049124108673));
#21487=CARTESIAN_POINT('Ctrl Pts',(242.031625185487,155.239682567333,244.684046451652));
#21488=CARTESIAN_POINT('Ctrl Pts',(241.898380736007,155.472987373266,244.573116753661));
#21489=CARTESIAN_POINT('Ctrl Pts',(241.704224565777,155.65704992868,244.573619803768));
#21490=CARTESIAN_POINT('Ctrl Pts',(242.051749888954,156.021528794222,244.070014088572));
#21491=CARTESIAN_POINT('Ctrl Pts',(241.718234113437,156.338315834566,244.070770482515));
#21492=CARTESIAN_POINT('Ctrl Pts',(241.338489677445,156.581146969436,244.236602955261));
#21493=CARTESIAN_POINT('Ctrl Pts',(240.743859410108,156.868106208125,244.785572840259));
#21494=CARTESIAN_POINT('Ctrl Pts',(240.540094008181,156.928680846509,245.174179737123));
#21495=CARTESIAN_POINT('Ctrl Pts',(240.541446108007,156.928221627357,245.975068211741));
#21496=CARTESIAN_POINT('Ctrl Pts',(240.744396066514,156.867920564623,246.361806700368));
#21497=CARTESIAN_POINT('Ctrl Pts',(241.339235998406,156.58070622062,246.911580897118));
#21498=CARTESIAN_POINT('Ctrl Pts',(241.719963975899,156.33710291391,247.077077359117));
#21499=CARTESIAN_POINT('Ctrl Pts',(242.387250650439,155.702410355244,247.077263646609));
#21500=CARTESIAN_POINT('Ctrl Pts',(242.645427060325,155.334768929497,246.910599101822));
#21501=CARTESIAN_POINT('Ctrl Pts',(242.959181374525,154.755791378006,246.361059656098));
#21502=CARTESIAN_POINT('Ctrl Pts',(243.029858527513,154.554695114521,245.972232660372));
#21503=CARTESIAN_POINT('Ctrl Pts',(243.029260143558,154.556159389752,245.171288638899));
#21504=CARTESIAN_POINT('Ctrl Pts',(242.958703359359,154.756718137498,244.784991571802));
#21505=CARTESIAN_POINT('Ctrl Pts',(242.644943159656,155.335595609506,244.23605360463));
#21506=CARTESIAN_POINT('Ctrl Pts',(242.385265664471,155.704741753878,244.06925769463));
#21507=CARTESIAN_POINT('Ctrl Pts',(242.051749888954,156.021528794222,244.070014088572));
#21508=CARTESIAN_POINT('',(241.704241838302,155.657068046185,246.573593133381));
#21509=CARTESIAN_POINT('',(241.704242970102,155.657069230833,244.573593133703));
#21510=CARTESIAN_POINT('Ctrl Pts',(241.704241838524,155.657068046418,246.573593133703));
#21511=CARTESIAN_POINT('Ctrl Pts',(241.736872664963,155.626024791641,246.573593133777));
#21512=CARTESIAN_POINT('Ctrl Pts',(241.767882349574,155.59363497048,246.570551147));
#21513=CARTESIAN_POINT('Ctrl Pts',(241.826534715335,155.526925812411,246.558577698866));
#21514=CARTESIAN_POINT('Ctrl Pts',(241.854090414984,155.492712431425,246.549670593028));
#21515=CARTESIAN_POINT('Ctrl Pts',(241.931937847661,155.387937570196,246.514389597396));
#21516=CARTESIAN_POINT('Ctrl Pts',(241.976284330344,155.316540049691,246.47971112174));
#21517=CARTESIAN_POINT('Ctrl Pts',(242.038432360623,155.199911928688,246.405940491082));
#21518=CARTESIAN_POINT('Ctrl Pts',(242.060099761803,155.153899400574,246.372086195779));
#21519=CARTESIAN_POINT('Ctrl Pts',(242.089421604343,155.084219718394,246.313003139576));
#21520=CARTESIAN_POINT('Ctrl Pts',(242.099060009831,155.059307245471,246.290206730024));
#21521=CARTESIAN_POINT('Ctrl Pts',(242.116743454559,155.011184520392,246.242334167609));
#21522=CARTESIAN_POINT('Ctrl Pts',(242.124923515658,154.987810179667,246.216956137048));
#21523=CARTESIAN_POINT('Ctrl Pts',(242.146344100199,154.92364651811,246.140681005568));
#21524=CARTESIAN_POINT('Ctrl Pts',(242.157701589958,154.885595585108,246.086958711194));
#21525=CARTESIAN_POINT('Ctrl Pts',(242.174748890245,154.822521444716,245.978032102338));
#21526=CARTESIAN_POINT('Ctrl Pts',(242.180851754483,154.796652641199,245.923416774259));
#21527=CARTESIAN_POINT('Ctrl Pts',(242.192502243845,154.741829624733,245.772513348259));
#21528=CARTESIAN_POINT('Ctrl Pts',(242.19491685745,154.722482122952,245.673483077984));
#21529=CARTESIAN_POINT('Ctrl Pts',(242.194939339411,154.722662003917,245.473008288348));
#21530=CARTESIAN_POINT('Ctrl Pts',(242.192458196941,154.74191321076,245.374193081089));
#21531=CARTESIAN_POINT('Ctrl Pts',(242.18073855789,154.796791362237,245.223303692942));
#21532=CARTESIAN_POINT('Ctrl Pts',(242.174629050872,154.822651099648,245.16876516982));
#21533=CARTESIAN_POINT('Ctrl Pts',(242.15759229929,154.885742196139,245.059926304006));
#21534=CARTESIAN_POINT('Ctrl Pts',(242.146250544142,154.92382744045,245.006226072546));
#21535=CARTESIAN_POINT('Ctrl Pts',(242.124835141528,154.988050584937,244.929954836604));
#21536=CARTESIAN_POINT('Ctrl Pts',(242.116647203304,155.011461461694,244.904560232997));
#21537=CARTESIAN_POINT('Ctrl Pts',(242.098943859986,155.059603438356,244.856699719665));
#21538=CARTESIAN_POINT('Ctrl Pts',(242.089314088538,155.084472314344,244.833955999992));
#21539=CARTESIAN_POINT('Ctrl Pts',(242.060018432519,155.154093511846,244.774957037284));
#21540=CARTESIAN_POINT('Ctrl Pts',(242.038370261862,155.200086959791,244.741137633888));
#21541=CARTESIAN_POINT('Ctrl Pts',(241.976228876202,155.316724936344,244.667392469806));
#21542=CARTESIAN_POINT('Ctrl Pts',(241.931856584362,155.388139210515,244.632719291294));
#21543=CARTESIAN_POINT('Ctrl Pts',(241.853959577504,155.492909761618,244.597463836825));
#21544=CARTESIAN_POINT('Ctrl Pts',(241.826400985401,155.527101906926,244.588569745954));
#21545=CARTESIAN_POINT('Ctrl Pts',(241.767780801273,155.593738280963,244.576624852807));
#21546=CARTESIAN_POINT('Ctrl Pts',(241.736817627638,155.626071525356,244.573593133703));
#21547=CARTESIAN_POINT('Ctrl Pts',(241.704242970102,155.657069230833,244.573593133703));
#21548=CARTESIAN_POINT('',(242.049277846445,156.018936140718,247.073589514835));
#21549=CARTESIAN_POINT('',(241.704240380882,155.657066517399,246.573591021215));
#21550=CARTESIAN_POINT('',(242.049280067237,156.018938485669,244.073593137428));
#21551=CARTESIAN_POINT('Ctrl Pts',(242.04928006672,156.018938485126,244.073593133703));
#21552=CARTESIAN_POINT('Ctrl Pts',(242.219085177029,155.857031770043,244.073325863255));
#21553=CARTESIAN_POINT('Ctrl Pts',(242.363945625518,155.690456210395,244.109847139091));
#21554=CARTESIAN_POINT('Ctrl Pts',(242.548946094757,155.444153214881,244.219811905837));
#21555=CARTESIAN_POINT('Ctrl Pts',(242.605251765288,155.362612438805,244.265663970251));
#21556=CARTESIAN_POINT('Ctrl Pts',(242.708167559415,155.202029405512,244.37576238341));
#21557=CARTESIAN_POINT('Ctrl Pts',(242.753983429964,155.124439488524,244.438626167558));
#21558=CARTESIAN_POINT('Ctrl Pts',(242.883294398959,154.888388370452,244.663127176969));
#21559=CARTESIAN_POINT('Ctrl Pts',(242.937958626695,154.765039089602,244.826245103114));
#21560=CARTESIAN_POINT('Ctrl Pts',(243.008010283782,154.599423235233,245.17938212848));
#21561=CARTESIAN_POINT('Ctrl Pts',(243.023489700801,154.556974142855,245.369501892319));
#21562=CARTESIAN_POINT('Ctrl Pts',(243.023766909856,154.556251500951,245.776239362339));
#21563=CARTESIAN_POINT('Ctrl Pts',(243.008413092906,154.598417281956,245.966395214971));
#21564=CARTESIAN_POINT('Ctrl Pts',(242.955809418766,154.722862723227,246.231809670352));
#21565=CARTESIAN_POINT('Ctrl Pts',(242.93321176695,154.774491255809,246.316977934885));
#21566=CARTESIAN_POINT('Ctrl Pts',(242.889789275449,154.866206518623,246.439775500791));
#21567=CARTESIAN_POINT('Ctrl Pts',(242.873719911226,154.899151839497,246.479882217612));
#21568=CARTESIAN_POINT('Ctrl Pts',(242.837984377284,154.969559473606,246.558444040955));
#21569=CARTESIAN_POINT('Ctrl Pts',(242.817773280998,155.008015020619,246.597842459808));
#21570=CARTESIAN_POINT('Ctrl Pts',(242.627600826482,155.354975670536,246.927734975046));
#21571=CARTESIAN_POINT('Ctrl Pts',(242.389986925115,155.694079425826,247.074098313406));
#21572=CARTESIAN_POINT('Ctrl Pts',(242.049278403401,156.018936725024,247.073589666413));
#21573=CARTESIAN_POINT('',(241.704242970102,155.657069230833,244.573593133703));
#21574=CARTESIAN_POINT('Ctrl Pts',(236.873741527621,150.590918454637,244.573619803768));
#21575=CARTESIAN_POINT('Ctrl Pts',(237.06789769785,150.406855899223,244.574122853875));
#21576=CARTESIAN_POINT('Ctrl Pts',(237.306163156749,150.283922676462,244.684411798912));
#21577=CARTESIAN_POINT('Ctrl Pts',(237.692910214852,150.159954573134,245.049510693237));
#21578=CARTESIAN_POINT('Ctrl Pts',(237.83095777893,150.145221417902,245.307955179719));
#21579=CARTESIAN_POINT('Ctrl Pts',(237.830050114206,150.145361269005,245.84060223374));
#21580=CARTESIAN_POINT('Ctrl Pts',(237.692550494078,150.1600125492,246.097804076277));
#21581=CARTESIAN_POINT('Ctrl Pts',(237.305689488997,150.28413750065,246.463437960953));
#21582=CARTESIAN_POINT('Ctrl Pts',(237.066827268937,150.407494951768,246.573503411772));
#21583=CARTESIAN_POINT('Ctrl Pts',(236.678495648654,150.776403597648,246.573627286256));
#21584=CARTESIAN_POINT('Ctrl Pts',(236.546112873865,151.008822575015,246.462784974605));
#21585=CARTESIAN_POINT('Ctrl Pts',(236.404536491293,151.388432970342,246.097307277076));
#21586=CARTESIAN_POINT('Ctrl Pts',(236.382973712424,151.525880629227,245.8387163343));
#21587=CARTESIAN_POINT('Ctrl Pts',(236.383191101889,151.524892037994,245.306032501962));
#21588=CARTESIAN_POINT('Ctrl Pts',(236.404745663322,151.387821786076,245.049124108673));
#21589=CARTESIAN_POINT('Ctrl Pts',(236.546340907911,151.008285815983,244.684046451652));
#21590=CARTESIAN_POINT('Ctrl Pts',(236.679585357392,150.774981010051,244.573116753661));
#21591=CARTESIAN_POINT('Ctrl Pts',(236.873741527621,150.590918454637,244.573619803768));
#21592=CARTESIAN_POINT('Ctrl Pts',(236.526170038182,150.226391170675,244.069947188143));
#21593=CARTESIAN_POINT('Ctrl Pts',(236.859704326629,149.909586498829,244.07070361574));
#21594=CARTESIAN_POINT('Ctrl Pts',(237.239467557095,149.666739436376,244.236543467048));
#21595=CARTESIAN_POINT('Ctrl Pts',(237.834125440234,149.379758545477,244.785537777997));
#21596=CARTESIAN_POINT('Ctrl Pts',(238.037899572308,149.319177817379,245.174161966009));
#21597=CARTESIAN_POINT('Ctrl Pts',(238.036547413442,149.319637078956,245.975086074588));
#21598=CARTESIAN_POINT('Ctrl Pts',(237.833588760324,149.379944205939,246.361841771235));
#21599=CARTESIAN_POINT('Ctrl Pts',(237.238721199914,149.667180215205,246.911640429713));
#21600=CARTESIAN_POINT('Ctrl Pts',(236.857974376567,149.91079949572,247.077144255326));
#21601=CARTESIAN_POINT('Ctrl Pts',(236.190650644836,150.545527361884,247.07733055111));
#21602=CARTESIAN_POINT('Ctrl Pts',(235.932457524162,150.913186750969,246.910658590737));
#21603=CARTESIAN_POINT('Ctrl Pts',(235.61868033735,151.492190786966,246.361094693722));
#21604=CARTESIAN_POINT('Ctrl Pts',(235.547996659869,151.693295505715,245.972250397064));
#21605=CARTESIAN_POINT('Ctrl Pts',(235.548595094435,151.691831167293,245.171270739137));
#21606=CARTESIAN_POINT('Ctrl Pts',(235.619158388231,151.491263985552,244.784956483677));
#21607=CARTESIAN_POINT('Ctrl Pts',(235.932941458821,150.912360032447,244.235994091974));
#21608=CARTESIAN_POINT('Ctrl Pts',(236.192635749735,150.543195842521,244.069190760545));
#21609=CARTESIAN_POINT('Ctrl Pts',(236.526170038182,150.226391170675,244.069947188143));
#21610=CARTESIAN_POINT('',(236.873724255103,150.590900337126,246.573593133381));
#21611=CARTESIAN_POINT('',(236.873723123297,150.590899152483,244.573593133703));
#21612=CARTESIAN_POINT('Ctrl Pts',(236.873724254881,150.590900336893,246.573593133703));
#21613=CARTESIAN_POINT('Ctrl Pts',(236.84109342844,150.621943591671,246.573593133777));
#21614=CARTESIAN_POINT('Ctrl Pts',(236.810083743827,150.654333412834,246.570551147));
#21615=CARTESIAN_POINT('Ctrl Pts',(236.751431378063,150.721042570906,246.558577698866));
#21616=CARTESIAN_POINT('Ctrl Pts',(236.723875678414,150.755255951892,246.549670593028));
#21617=CARTESIAN_POINT('Ctrl Pts',(236.646028245737,150.860030813121,246.514389597396));
#21618=CARTESIAN_POINT('Ctrl Pts',(236.601681763054,150.931428333627,246.47971112174));
#21619=CARTESIAN_POINT('Ctrl Pts',(236.539533732776,151.048056454629,246.405940491082));
#21620=CARTESIAN_POINT('Ctrl Pts',(236.517866331595,151.094068982743,246.372086195779));
#21621=CARTESIAN_POINT('Ctrl Pts',(236.488544489055,151.163748664924,246.313003139575));
#21622=CARTESIAN_POINT('Ctrl Pts',(236.478906083567,151.188661137847,246.290206730023));
#21623=CARTESIAN_POINT('Ctrl Pts',(236.461222638839,151.236783862925,246.242334167609));
#21624=CARTESIAN_POINT('Ctrl Pts',(236.453042577741,151.26015820365,246.216956137048));
#21625=CARTESIAN_POINT('Ctrl Pts',(236.431621993199,151.324321865207,246.140681005568));
#21626=CARTESIAN_POINT('Ctrl Pts',(236.42026450344,151.362372798209,246.086958711194));
#21627=CARTESIAN_POINT('Ctrl Pts',(236.403217203154,151.4254469386,245.978032102337));
#21628=CARTESIAN_POINT('Ctrl Pts',(236.397114338915,151.451315742117,245.923416774258));
#21629=CARTESIAN_POINT('Ctrl Pts',(236.385463849553,151.506138758584,245.772513348258));
#21630=CARTESIAN_POINT('Ctrl Pts',(236.383049235948,151.525486260365,245.673483077983));
#21631=CARTESIAN_POINT('Ctrl Pts',(236.383026753987,151.5253063794,245.473008288348));
#21632=CARTESIAN_POINT('Ctrl Pts',(236.385507896457,151.506055172556,245.374193081089));
#21633=CARTESIAN_POINT('Ctrl Pts',(236.397227535509,151.45117702108,245.223303692942));
#21634=CARTESIAN_POINT('Ctrl Pts',(236.403337042526,151.425317283669,245.16876516982));
#21635=CARTESIAN_POINT('Ctrl Pts',(236.420373794109,151.362226187178,245.059926304005));
#21636=CARTESIAN_POINT('Ctrl Pts',(236.431715549256,151.324140942867,245.006226072545));
#21637=CARTESIAN_POINT('Ctrl Pts',(236.45313095187,151.25991779838,244.929954836604));
#21638=CARTESIAN_POINT('Ctrl Pts',(236.461318890094,151.236506921622,244.904560232997));
#21639=CARTESIAN_POINT('Ctrl Pts',(236.479022233412,151.188364944961,244.856699719665));
#21640=CARTESIAN_POINT('Ctrl Pts',(236.488652004861,151.163496068973,244.833955999992));
#21641=CARTESIAN_POINT('Ctrl Pts',(236.517947660879,151.09387487147,244.774957037284));
#21642=CARTESIAN_POINT('Ctrl Pts',(236.539595831537,151.047881423526,244.741137633888));
#21643=CARTESIAN_POINT('Ctrl Pts',(236.601737217197,150.931243446973,244.667392469806));
#21644=CARTESIAN_POINT('Ctrl Pts',(236.646109509036,150.859829172802,244.632719291294));
#21645=CARTESIAN_POINT('Ctrl Pts',(236.724006515894,150.755058621699,244.597463836825));
#21646=CARTESIAN_POINT('Ctrl Pts',(236.751565107997,150.720866476391,244.588569745954));
#21647=CARTESIAN_POINT('Ctrl Pts',(236.810185292125,150.654230102354,244.576624852807));
#21648=CARTESIAN_POINT('Ctrl Pts',(236.841148465761,150.621896857961,244.573593133703));
#21649=CARTESIAN_POINT('Ctrl Pts',(236.873723123297,150.590899152483,244.573593133703));
#21650=CARTESIAN_POINT('',(236.528689854778,150.229030713486,247.073589202258));
#21651=CARTESIAN_POINT('',(236.873725712516,150.590901865917,246.573591021215));
#21652=CARTESIAN_POINT('',(236.528686026161,150.229029897647,244.073593137428));
#21653=CARTESIAN_POINT('Ctrl Pts',(236.528686026679,150.229029898191,244.073593133703));
#21654=CARTESIAN_POINT('Ctrl Pts',(236.358977792143,150.390844243626,244.073207336743));
#21655=CARTESIAN_POINT('Ctrl Pts',(236.214147012029,150.557360059161,244.109671982816));
#21656=CARTESIAN_POINT('Ctrl Pts',(236.029129074192,150.80366177929,244.219644650044));
#21657=CARTESIAN_POINT('Ctrl Pts',(235.972807292529,150.88521660712,244.26551482214));
#21658=CARTESIAN_POINT('Ctrl Pts',(235.86984508284,151.045860635605,244.375680399037));
#21659=CARTESIAN_POINT('Ctrl Pts',(235.823963573414,151.123561960789,244.438654405421));
#21660=CARTESIAN_POINT('Ctrl Pts',(235.694654847654,151.359614330903,244.663166238249));
#21661=CARTESIAN_POINT('Ctrl Pts',(235.639993226236,151.482961305671,244.826292334005));
#21662=CARTESIAN_POINT('Ctrl Pts',(235.569947693597,151.648565991774,245.179447606592));
#21663=CARTESIAN_POINT('Ctrl Pts',(235.554471743642,151.691006359538,245.369584971744));
#21664=CARTESIAN_POINT('Ctrl Pts',(235.554203716487,151.691705065711,245.776329368437));
#21665=CARTESIAN_POINT('Ctrl Pts',(235.569563174184,151.649524262202,245.966487747264));
#21666=CARTESIAN_POINT('Ctrl Pts',(235.622179572538,151.525052876751,246.231904586228));
#21667=CARTESIAN_POINT('Ctrl Pts',(235.644782194467,151.473415137899,246.317073411003));
#21668=CARTESIAN_POINT('Ctrl Pts',(235.688213704026,151.381685522078,246.439871465846));
#21669=CARTESIAN_POINT('Ctrl Pts',(235.704286335514,151.348735327601,246.479978287074));
#21670=CARTESIAN_POINT('Ctrl Pts',(235.740029011678,151.278317835617,246.55854020209));
#21671=CARTESIAN_POINT('Ctrl Pts',(235.760244184763,151.239857072587,246.597938651966));
#21672=CARTESIAN_POINT('Ctrl Pts',(235.950439876362,150.892877130181,246.927807707392));
#21673=CARTESIAN_POINT('Ctrl Pts',(236.187731957931,150.554124308018,247.074228761836));
#21674=CARTESIAN_POINT('Ctrl Pts',(236.528689297355,150.229030128645,247.073589199254));
#21675=CARTESIAN_POINT('',(236.873723123297,150.590899152483,244.573593133703));
#21676=CARTESIAN_POINT('Origin',(242.04928006672,156.018938485126,245.573593133703));
#21677=CARTESIAN_POINT('Ctrl Pts',(241.704242970102,155.657069230833,244.573593133703));
#21678=CARTESIAN_POINT('Ctrl Pts',(241.630962824868,155.726801855244,244.573593133703));
#21679=CARTESIAN_POINT('Ctrl Pts',(241.551605382331,155.78805678601,244.588926668372));
#21680=CARTESIAN_POINT('Ctrl Pts',(241.443050901967,155.858045218471,244.628234491494));
#21681=CARTESIAN_POINT('Ctrl Pts',(241.415780822802,155.874503493771,244.639604524938));
#21682=CARTESIAN_POINT('Ctrl Pts',(241.272162238111,155.955893693544,244.707242077006));
#21683=CARTESIAN_POINT('Ctrl Pts',(241.164964889003,155.998554010553,244.784746950616));
#21684=CARTESIAN_POINT('Ctrl Pts',(241.063791249207,156.030721162401,244.880838247272));
#21685=CARTESIAN_POINT('Ctrl Pts',(241.051524170799,156.034520712982,244.89301514354));
#21686=CARTESIAN_POINT('Ctrl Pts',(241.02744274686,156.041789826092,244.918011816567));
#21687=CARTESIAN_POINT('Ctrl Pts',(241.015630708891,156.045257826393,244.930834103936));
#21688=CARTESIAN_POINT('Ctrl Pts',(240.960645876954,156.06096670119,244.993308664963));
#21689=CARTESIAN_POINT('Ctrl Pts',(240.921101198906,156.070922047133,245.04672122124));
#21690=CARTESIAN_POINT('Ctrl Pts',(240.855267036901,156.085703737406,245.155343526424));
#21691=CARTESIAN_POINT('Ctrl Pts',(240.82813302031,156.090901164723,245.20995619415));
#21692=CARTESIAN_POINT('Ctrl Pts',(240.786741009928,156.097888240926,245.317836348554));
#21693=CARTESIAN_POINT('Ctrl Pts',(240.771507778469,156.099964606954,245.37057049282));
#21694=CARTESIAN_POINT('Ctrl Pts',(240.752244886547,156.102294553641,245.473637636456));
#21695=CARTESIAN_POINT('Ctrl Pts',(240.747419389518,156.102688907628,245.52350987106));
#21696=CARTESIAN_POINT('Ctrl Pts',(240.747508336191,156.102780888958,245.66744290748));
#21697=CARTESIAN_POINT('Ctrl Pts',(240.764538417831,156.101609329828,245.766443228677));
#21698=CARTESIAN_POINT('Ctrl Pts',(240.822244927711,156.092107051219,245.923804651633));
#21699=CARTESIAN_POINT('Ctrl Pts',(240.848360549117,156.087222664751,245.978365805299));
#21700=CARTESIAN_POINT('Ctrl Pts',(240.912182483255,156.073188120536,246.087229534118));
#21701=CARTESIAN_POINT('Ctrl Pts',(240.95075681251,156.063667434727,246.140929653169));
#21702=CARTESIAN_POINT('Ctrl Pts',(241.01592973934,156.045337831578,246.21720597302));
#21703=CARTESIAN_POINT('Ctrl Pts',(241.039710474856,156.038276122433,246.242605470456));
#21704=CARTESIAN_POINT('Ctrl Pts',(241.08864266278,156.022897012116,246.290460601381));
#21705=CARTESIAN_POINT('Ctrl Pts',(241.11395054769,156.014462688202,246.313212577001));
#21706=CARTESIAN_POINT('Ctrl Pts',(241.184850160234,155.988500534368,246.372197845411));
#21707=CARTESIAN_POINT('Ctrl Pts',(241.231762406002,155.969048729803,246.406000105603));
#21708=CARTESIAN_POINT('Ctrl Pts',(241.315513812164,155.929351171955,246.457744032173));
#21709=CARTESIAN_POINT('Ctrl Pts',(241.351844268562,155.910582668646,246.477508148981));
#21710=CARTESIAN_POINT('Ctrl Pts',(241.415584476112,155.874491292809,246.507530839585));
#21711=CARTESIAN_POINT('Ctrl Pts',(241.442873673692,155.858037293914,246.518909668632));
#21712=CARTESIAN_POINT('Ctrl Pts',(241.551506550977,155.78806465653,246.558247879177));
#21713=CARTESIAN_POINT('Ctrl Pts',(241.630918492936,155.726824027084,246.573593133538));
#21714=CARTESIAN_POINT('Ctrl Pts',(241.704241838524,155.657068046418,246.573593133703));
#21715=CARTESIAN_POINT('',(242.04928006672,156.018938485126,246.573593133703));
#21716=CARTESIAN_POINT('Ctrl Pts',(236.873723123297,150.590899152483,244.573593133703));
#21717=CARTESIAN_POINT('Ctrl Pts',(236.94700326853,150.521166528072,244.573593133703));
#21718=CARTESIAN_POINT('Ctrl Pts',(237.026360711067,150.459911597307,244.588926668372));
#21719=CARTESIAN_POINT('Ctrl Pts',(237.134915191431,150.389923164846,244.628234491494));
#21720=CARTESIAN_POINT('Ctrl Pts',(237.162185270595,150.373464889546,244.639604524937));
#21721=CARTESIAN_POINT('Ctrl Pts',(237.305803855289,150.292074689772,244.707242077007));
#21722=CARTESIAN_POINT('Ctrl Pts',(237.413001204397,150.249414372764,244.784746950618));
#21723=CARTESIAN_POINT('Ctrl Pts',(237.514174844192,150.217247220916,244.880838247272));
#21724=CARTESIAN_POINT('Ctrl Pts',(237.526441922599,150.213447670335,244.89301514354));
#21725=CARTESIAN_POINT('Ctrl Pts',(237.550523346536,150.206178557225,244.918011816565));
#21726=CARTESIAN_POINT('Ctrl Pts',(237.562335384507,150.202710556923,244.930834103935));
#21727=CARTESIAN_POINT('Ctrl Pts',(237.617320216445,150.187001682126,244.993308664963));
#21728=CARTESIAN_POINT('Ctrl Pts',(237.656864894493,150.177046336184,245.046721221241));
#21729=CARTESIAN_POINT('Ctrl Pts',(237.722699056497,150.162264645911,245.155343526424));
#21730=CARTESIAN_POINT('Ctrl Pts',(237.749833073088,150.157067218594,245.20995619415));
#21731=CARTESIAN_POINT('Ctrl Pts',(237.79122508347,150.150080142391,245.317836348554));
#21732=CARTESIAN_POINT('Ctrl Pts',(237.80645831493,150.148003776363,245.37057049282));
#21733=CARTESIAN_POINT('Ctrl Pts',(237.825721206852,150.145673829676,245.473637636457));
#21734=CARTESIAN_POINT('Ctrl Pts',(237.83054670388,150.145279475689,245.52350987106));
#21735=CARTESIAN_POINT('Ctrl Pts',(237.830457757208,150.145187494359,245.667442907476));
#21736=CARTESIAN_POINT('Ctrl Pts',(237.813427675569,150.146359053489,245.766443228673));
#21737=CARTESIAN_POINT('Ctrl Pts',(237.755721165688,150.155861332098,245.923804651633));
#21738=CARTESIAN_POINT('Ctrl Pts',(237.729605544281,150.160745718566,245.978365805299));
#21739=CARTESIAN_POINT('Ctrl Pts',(237.665783610144,150.17478026278,246.087229534118));
#21740=CARTESIAN_POINT('Ctrl Pts',(237.627209280889,150.18430094859,246.140929653169));
#21741=CARTESIAN_POINT('Ctrl Pts',(237.562036354058,150.202630551739,246.21720597302));
#21742=CARTESIAN_POINT('Ctrl Pts',(237.538255618541,150.209692260884,246.242605470456));
#21743=CARTESIAN_POINT('Ctrl Pts',(237.489323430618,150.225071371201,246.290460601382));
#21744=CARTESIAN_POINT('Ctrl Pts',(237.464015545708,150.233505695115,246.313212577001));
#21745=CARTESIAN_POINT('Ctrl Pts',(237.393115933165,150.259467848949,246.372197845411));
#21746=CARTESIAN_POINT('Ctrl Pts',(237.346203687396,150.278919653514,246.406000105603));
#21747=CARTESIAN_POINT('Ctrl Pts',(237.262452281233,150.318617211362,246.457744032174));
#21748=CARTESIAN_POINT('Ctrl Pts',(237.226121824836,150.337385714671,246.477508148981));
#21749=CARTESIAN_POINT('Ctrl Pts',(237.162381617287,150.373477090508,246.507530839585));
#21750=CARTESIAN_POINT('Ctrl Pts',(237.135092419706,150.389931089402,246.518909668632));
#21751=CARTESIAN_POINT('Ctrl Pts',(237.026459542421,150.459903726787,246.558247879178));
#21752=CARTESIAN_POINT('Ctrl Pts',(236.947047600469,150.521144356227,246.573593133537));
#21753=CARTESIAN_POINT('Ctrl Pts',(236.873724254881,150.590900336893,246.573593133703));
#21754=CARTESIAN_POINT('Origin',(239.288983046699,153.123984191658,244.073593133703));
#21755=CARTESIAN_POINT('Origin',(239.288983046699,153.123984191658,244.073593133703));
#21756=CARTESIAN_POINT('',(241.252450952944,155.183237164813,242.073593133703));
#21757=CARTESIAN_POINT('',(242.04928006672,156.018938485126,244.073593133703));
#21758=CARTESIAN_POINT('Origin',(239.288983046699,153.123984191658,242.073593133703));
#21759=CARTESIAN_POINT('Origin',(239.288983046699,153.123984191658,244.073593133703));
#21760=CARTESIAN_POINT('Origin',(239.288983046699,153.123984191658,275.073593133703));
#21761=CARTESIAN_POINT('',(242.04928006672,156.018938485126,271.473593133703));
#21762=CARTESIAN_POINT('Origin',(239.288983046699,153.123984191658,271.473593133703));
#21763=CARTESIAN_POINT('',(242.04928006672,156.018938485126,275.073593133703));
#21764=CARTESIAN_POINT('Ctrl Pts',(242.049278403401,156.018936725024,247.073589666413));
#21765=CARTESIAN_POINT('Ctrl Pts',(241.879080979887,156.181220851564,247.073336255209));
#21766=CARTESIAN_POINT('Ctrl Pts',(241.70548469323,156.318159568681,247.036490765957));
#21767=CARTESIAN_POINT('Ctrl Pts',(241.450419954028,156.491290181965,246.926335097092));
#21768=CARTESIAN_POINT('Ctrl Pts',(241.366251820411,156.543639888291,246.880468634973));
#21769=CARTESIAN_POINT('Ctrl Pts',(241.200961977391,156.638728451252,246.770439899073));
#21770=CARTESIAN_POINT('Ctrl Pts',(241.121296005925,156.68075993574,246.707630692229));
#21771=CARTESIAN_POINT('Ctrl Pts',(240.879699838575,156.798452586541,246.48357204053));
#21772=CARTESIAN_POINT('Ctrl Pts',(240.754085054325,156.847092028425,246.320599865048));
#21773=CARTESIAN_POINT('Ctrl Pts',(240.585611844582,156.909061419067,245.967456032054));
#21774=CARTESIAN_POINT('Ctrl Pts',(240.542567166162,156.922474283323,245.777012017024));
#21775=CARTESIAN_POINT('Ctrl Pts',(240.541906382068,156.922692292675,245.370016379345));
#21776=CARTESIAN_POINT('Ctrl Pts',(240.584720718821,156.909371480944,245.179908713947));
#21777=CARTESIAN_POINT('Ctrl Pts',(240.711375508263,156.862810604652,244.914832446015));
#21778=CARTESIAN_POINT('Ctrl Pts',(240.763953172911,156.842724194531,244.829821228398));
#21779=CARTESIAN_POINT('Ctrl Pts',(240.857506848798,156.803776862828,244.707325709514));
#21780=CARTESIAN_POINT('Ctrl Pts',(240.891134475151,156.789317054963,244.667330754476));
#21781=CARTESIAN_POINT('Ctrl Pts',(240.963066033618,156.757027041863,244.58901461358));
#21782=CARTESIAN_POINT('Ctrl Pts',(241.002349559882,156.738719066925,244.549787659307));
#21783=CARTESIAN_POINT('Ctrl Pts',(241.358027470615,156.565316622201,244.220670026599));
#21784=CARTESIAN_POINT('Ctrl Pts',(241.709462908565,156.342949227238,244.074128067476));
#21785=CARTESIAN_POINT('Ctrl Pts',(242.04928006672,156.018938485126,244.073593133703));
#21786=CARTESIAN_POINT('Ctrl Pts',(236.528689297355,150.229030128645,247.073589199254));
#21787=CARTESIAN_POINT('Ctrl Pts',(236.698998928806,150.066639190825,247.073269716825));
#21788=CARTESIAN_POINT('Ctrl Pts',(236.872669356512,149.92966652065,247.036390577158));
#21789=CARTESIAN_POINT('Ctrl Pts',(237.127746428412,149.756549620958,246.926232368273));
#21790=CARTESIAN_POINT('Ctrl Pts',(237.21190246902,149.704215227193,246.880373048748));
#21791=CARTESIAN_POINT('Ctrl Pts',(237.335824368256,149.632932480362,246.797874194614));
#21792=CARTESIAN_POINT('Ctrl Pts',(237.376748308819,149.610374208359,246.768089597428));
#21793=CARTESIAN_POINT('Ctrl Pts',(237.457684600991,149.567519259982,246.703950444775));
#21794=CARTESIAN_POINT('Ctrl Pts',(237.496910490698,149.547605679369,246.670325582074));
#21795=CARTESIAN_POINT('Ctrl Pts',(237.698299988104,149.449498601363,246.483479342273));
#21796=CARTESIAN_POINT('Ctrl Pts',(237.823942114196,149.400852263453,246.320448669587));
#21797=CARTESIAN_POINT('Ctrl Pts',(237.992420893058,149.338884077992,245.967279962524));
#21798=CARTESIAN_POINT('Ctrl Pts',(238.03544226452,149.325479801998,245.776985842833));
#21799=CARTESIAN_POINT('Ctrl Pts',(238.036014742284,149.325290926997,245.369914584485));
#21800=CARTESIAN_POINT('Ctrl Pts',(237.993179236838,149.338619575289,245.179793889859));
#21801=CARTESIAN_POINT('Ctrl Pts',(237.866527219159,149.385181894555,244.914735249744));
#21802=CARTESIAN_POINT('Ctrl Pts',(237.813956192467,149.405266919668,244.829736103342));
#21803=CARTESIAN_POINT('Ctrl Pts',(237.720420540777,149.444208076534,244.707267984196));
#21804=CARTESIAN_POINT('Ctrl Pts',(237.686800262615,149.458665134707,244.667283711223));
#21805=CARTESIAN_POINT('Ctrl Pts',(237.614885931005,149.490947953181,244.588992032097));
#21806=CARTESIAN_POINT('Ctrl Pts',(237.57558597426,149.509264161755,244.54975425391));
#21807=CARTESIAN_POINT('Ctrl Pts',(237.220147950135,149.682550133189,244.220906926231));
#21808=CARTESIAN_POINT('Ctrl Pts',(236.86867264184,149.904857581276,244.074366090943));
#21809=CARTESIAN_POINT('Ctrl Pts',(236.528686026679,150.229029898191,244.073593133703));
#21810=CARTESIAN_POINT('Origin',(239.288983046699,153.123984191658,271.473593133703));
#21811=CARTESIAN_POINT('',(242.463324619723,156.453181629146,272.073593133703));
#21812=CARTESIAN_POINT('Origin',(239.288983046699,153.123984191658,272.073593133703));
#21813=CARTESIAN_POINT('Origin',(242.463324619723,156.453181629146,271.473593133703));
#21814=CARTESIAN_POINT('Origin',(239.288983046699,153.123984191658,275.073593133703));
#21815=CARTESIAN_POINT('',(234.458463261663,148.05781417809,274.073593133703));
#21816=CARTESIAN_POINT('',(244.119502831735,158.190154205226,274.073593133703));
#21817=CARTESIAN_POINT('Origin',(239.288983046699,153.123984191658,274.073593133703));
#21818=CARTESIAN_POINT('Origin',(239.288983046699,153.123984191658,274.073593133703));
#21819=CARTESIAN_POINT('',(244.119502831735,158.190154205226,272.073593133703));
#21820=CARTESIAN_POINT('',(244.119502831735,158.190154205226,275.073593133703));
#21821=CARTESIAN_POINT('Origin',(239.288983046699,153.123984191658,272.073593133703));
#21822=CARTESIAN_POINT('Origin',(239.288983046699,153.123984191658,275.073593133703));
#21823=CARTESIAN_POINT('',(235.148537516668,148.781552751457,275.073593133703));
#21824=CARTESIAN_POINT('',(235.148537516668,148.781552751457,275.073593133703));
#21825=CARTESIAN_POINT('Origin',(239.288983046699,153.123984191658,275.073593133703));
#21826=CARTESIAN_POINT('Origin',(239.288983046699,153.123984191658,275.073593133703));
#21827=CARTESIAN_POINT('Origin',(244.355153060267,148.293464406622,272.073593133703));
#21828=CARTESIAN_POINT('Origin',(241.348236019854,151.160516285414,242.073593133703));
#21829=CARTESIAN_POINT('Ctrl Pts',(236.873740135465,150.590916994567,244.573617786368));
#21830=CARTESIAN_POINT('Ctrl Pts',(237.067896863957,150.406853907471,244.57412083749));
#21831=CARTESIAN_POINT('Ctrl Pts',(237.306162889608,150.283920204409,244.68441000503));
#21832=CARTESIAN_POINT('Ctrl Pts',(237.692910780473,150.159951448154,245.049509635926));
#21833=CARTESIAN_POINT('Ctrl Pts',(237.83095860781,150.145218109284,245.307954643826));
#21834=CARTESIAN_POINT('Ctrl Pts',(237.830050941306,150.145357961667,245.840602772399));
#21835=CARTESIAN_POINT('Ctrl Pts',(237.69255105899,150.160009424731,246.097805133848));
#21836=CARTESIAN_POINT('Ctrl Pts',(237.305689220764,150.284135029502,246.463439756173));
#21837=CARTESIAN_POINT('Ctrl Pts',(237.066826432402,150.407492962315,246.573505429044));
#21838=CARTESIAN_POINT('Ctrl Pts',(236.67849369465,150.776402672902,246.573629303778));
#21839=CARTESIAN_POINT('Ctrl Pts',(236.546110415943,151.008822191958,246.462786768509));
#21840=CARTESIAN_POINT('Ctrl Pts',(236.404533343642,151.388433385931,246.097308333644));
#21841=CARTESIAN_POINT('Ctrl Pts',(236.382970368025,151.525881299787,245.838716869155));
#21842=CARTESIAN_POINT('Ctrl Pts',(236.383187759016,151.524892706649,245.306031962191));
#21843=CARTESIAN_POINT('Ctrl Pts',(236.404742516748,151.387822200401,245.049123050581));
#21844=CARTESIAN_POINT('Ctrl Pts',(236.546338451014,151.008285431764,244.684044657033));
#21845=CARTESIAN_POINT('Ctrl Pts',(236.679583406974,150.774980081663,244.573114735247));
#21846=CARTESIAN_POINT('Ctrl Pts',(236.873740135465,150.590916994567,244.573617786368));
#21847=CARTESIAN_POINT('Ctrl Pts',(236.525220476937,150.225395286397,244.068571160446));
#21848=CARTESIAN_POINT('Ctrl Pts',(236.859135544773,149.908227964641,244.069328280267));
#21849=CARTESIAN_POINT('Ctrl Pts',(237.239285345497,149.66505329898,244.235319896002));
#21850=CARTESIAN_POINT('Ctrl Pts',(237.834511238579,149.377627059051,244.784816607079));
#21851=CARTESIAN_POINT('Ctrl Pts',(238.038464934868,149.31692107592,245.173796444513));
#21852=CARTESIAN_POINT('Ctrl Pts',(238.03711156165,149.317381210123,245.975453482869));
#21853=CARTESIAN_POINT('Ctrl Pts',(237.833974075219,149.377813068345,246.36256311913));
#21854=CARTESIAN_POINT('Ctrl Pts',(237.238538243332,149.665494695115,246.912864913618));
#21855=CARTESIAN_POINT('Ctrl Pts',(236.857403792907,149.909442529541,247.078520196222));
#21856=CARTESIAN_POINT('Ctrl Pts',(236.189317857989,150.544896610707,247.07870666254));
#21857=CARTESIAN_POINT('Ctrl Pts',(235.930781024921,150.912925475016,246.91188217622));
#21858=CARTESIAN_POINT('Ctrl Pts',(235.616533387526,151.492474252108,246.36181535786));
#21859=CARTESIAN_POINT('Ctrl Pts',(235.545715512323,151.6937528812,245.972615210562));
#21860=CARTESIAN_POINT('Ctrl Pts',(235.546314987901,151.692287243042,245.170902571576));
#21861=CARTESIAN_POINT('Ctrl Pts',(235.61701217298,151.491546588432,244.784234780814));
#21862=CARTESIAN_POINT('Ctrl Pts',(235.931265658698,150.912097964328,244.234770018165));
#21863=CARTESIAN_POINT('Ctrl Pts',(236.1913054091,150.542562608153,244.067814040624));
#21864=CARTESIAN_POINT('Ctrl Pts',(236.525220476937,150.225395286397,244.068571160446));
#21865=CARTESIAN_POINT('Ctrl Pts',(241.704225957933,155.65705138875,244.573617786368));
#21866=CARTESIAN_POINT('Ctrl Pts',(241.510069229442,155.841114475846,244.57412083749));
#21867=CARTESIAN_POINT('Ctrl Pts',(241.27180320379,155.964048178908,244.68441000503));
#21868=CARTESIAN_POINT('Ctrl Pts',(240.885055312925,156.088016935163,245.049509635926));
#21869=CARTESIAN_POINT('Ctrl Pts',(240.747007485588,156.102750274032,245.307954643826));
#21870=CARTESIAN_POINT('Ctrl Pts',(240.747915152092,156.102610421649,245.840602772399));
#21871=CARTESIAN_POINT('Ctrl Pts',(240.885415034409,156.087958958585,246.097805133848));
#21872=CARTESIAN_POINT('Ctrl Pts',(241.272276872634,155.963833353815,246.463439756173));
#21873=CARTESIAN_POINT('Ctrl Pts',(241.511139660996,155.840475421002,246.573505429044));
#21874=CARTESIAN_POINT('Ctrl Pts',(241.899472398749,155.471565710415,246.573629303778));
#21875=CARTESIAN_POINT('Ctrl Pts',(242.031855677455,155.239146191359,246.462786768509));
#21876=CARTESIAN_POINT('Ctrl Pts',(242.173432749756,154.859534997386,246.097308333644));
#21877=CARTESIAN_POINT('Ctrl Pts',(242.194995725373,154.72208708353,245.838716869155));
#21878=CARTESIAN_POINT('Ctrl Pts',(242.194778334383,154.723075676668,245.306031962191));
#21879=CARTESIAN_POINT('Ctrl Pts',(242.17322357665,154.860146182915,245.049123050581));
#21880=CARTESIAN_POINT('Ctrl Pts',(242.031627642384,155.239682951552,244.684044657033));
#21881=CARTESIAN_POINT('Ctrl Pts',(241.898382686424,155.472988301653,244.573114735247));
#21882=CARTESIAN_POINT('Ctrl Pts',(241.704225957933,155.65705138875,244.573617786368));
#21883=CARTESIAN_POINT('Ctrl Pts',(242.052768019306,156.022596592656,244.068538696047));
#21884=CARTESIAN_POINT('Ctrl Pts',(241.718843967803,156.339772470352,244.0692958322));
#21885=CARTESIAN_POINT('Ctrl Pts',(241.33868504679,156.582954865103,244.235291028488));
#21886=CARTESIAN_POINT('Ctrl Pts',(240.743445752741,156.870391612079,244.78479959261));
#21887=CARTESIAN_POINT('Ctrl Pts',(240.539487820023,156.931100550332,245.173787820824));
#21888=CARTESIAN_POINT('Ctrl Pts',(240.540841221892,156.930640395541,245.975462151073));
#21889=CARTESIAN_POINT('Ctrl Pts',(240.743982927508,156.870205594555,246.362580137774));
#21890=CARTESIAN_POINT('Ctrl Pts',(241.339432166532,156.582513454404,246.912893802668));
#21891=CARTESIAN_POINT('Ctrl Pts',(241.720575762179,156.338557868458,247.078552658573));
#21892=CARTESIAN_POINT('Ctrl Pts',(242.388679679633,155.703086653819,247.078739128914));
#21893=CARTESIAN_POINT('Ctrl Pts',(242.647224621851,155.335049072542,246.911911044074));
#21894=CARTESIAN_POINT('Ctrl Pts',(242.961483358511,154.755487443462,246.361832360372));
#21895=CARTESIAN_POINT('Ctrl Pts',(243.032304399819,154.554204711331,245.972623817548));
#21896=CARTESIAN_POINT('Ctrl Pts',(243.031704899681,154.555670380153,245.170893885459));
#21897=CARTESIAN_POINT('Ctrl Pts',(242.961004555727,154.756415127481,244.784217753795));
#21898=CARTESIAN_POINT('Ctrl Pts',(242.646739971581,155.33587660192,244.234741138791));
#21899=CARTESIAN_POINT('Ctrl Pts',(242.386692070809,155.705420714959,244.067781559894));
#21900=CARTESIAN_POINT('Ctrl Pts',(242.052768019306,156.022596592656,244.068538696047));
#21901=CARTESIAN_POINT('Ctrl Pts',(272.893594663547,160.159358297364,244.573616253716));
#21902=CARTESIAN_POINT('Ctrl Pts',(273.160746650237,160.173717428468,244.574119305608));
#21903=CARTESIAN_POINT('Ctrl Pts',(273.413857808985,160.262139317963,244.684408642187));
#21904=CARTESIAN_POINT('Ctrl Pts',(273.76983864822,160.457639798944,245.049508832668));
#21905=CARTESIAN_POINT('Ctrl Pts',(273.875476617283,160.547722831363,245.3079542367));
#21906=CARTESIAN_POINT('Ctrl Pts',(273.874750844349,160.547160093815,245.840603181627));
#21907=CARTESIAN_POINT('Ctrl Pts',(273.769549161884,160.45741853231,246.097805937303));
#21908=CARTESIAN_POINT('Ctrl Pts',(273.413376091047,160.261943203446,246.463441120033));
#21909=CARTESIAN_POINT('Ctrl Pts',(273.159546539055,160.173379857016,246.5735069616));
#21910=CARTESIAN_POINT('Ctrl Pts',(272.624660495995,160.145186473407,246.573630836524));
#21911=CARTESIAN_POINT('Ctrl Pts',(272.364888729948,160.208928826216,246.462788131368));
#21912=CARTESIAN_POINT('Ctrl Pts',(271.991939938556,160.367227701822,246.097309136337));
#21913=CARTESIAN_POINT('Ctrl Pts',(271.877329515132,160.446103563013,245.838717275493));
#21914=CARTESIAN_POINT('Ctrl Pts',(271.878196696175,160.445581475241,245.306031552117));
#21915=CARTESIAN_POINT('Ctrl Pts',(271.992527488176,160.36695920955,245.049122246731));
#21916=CARTESIAN_POINT('Ctrl Pts',(272.365435222693,160.208725212658,244.68404329363));
#21917=CARTESIAN_POINT('Ctrl Pts',(272.626442676856,160.14499916626,244.573113201823));
#21918=CARTESIAN_POINT('Ctrl Pts',(272.893594663547,160.159358297364,244.573616253716));
#21919=CARTESIAN_POINT('Ctrl Pts',(272.919178153013,159.656406407913,244.070014088572));
#21920=CARTESIAN_POINT('Ctrl Pts',(273.378524344086,159.680652607522,244.070770482515));
#21921=CARTESIAN_POINT('Ctrl Pts',(273.815975906659,159.789321495117,244.236602955261));
#21922=CARTESIAN_POINT('Ctrl Pts',(274.433249479638,160.023637725035,244.785572840259));
#21923=CARTESIAN_POINT('Ctrl Pts',(274.617362800752,160.129901128078,245.174179737123));
#21924=CARTESIAN_POINT('Ctrl Pts',(274.616099527232,160.129235398268,245.975068211741));
#21925=CARTESIAN_POINT('Ctrl Pts',(274.432745627596,160.023375815266,246.361806700368));
#21926=CARTESIAN_POINT('Ctrl Pts',(273.815142664649,159.789082827464,246.911580897118));
#21927=CARTESIAN_POINT('Ctrl Pts',(273.376454115703,159.680230997393,247.077077359117));
#21928=CARTESIAN_POINT('Ctrl Pts',(272.456774314034,159.632322621868,247.077263646609));
#21929=CARTESIAN_POINT('Ctrl Pts',(272.012324858108,159.697744007317,246.910599101822));
#21930=CARTESIAN_POINT('Ctrl Pts',(271.376232398275,159.868164538219,246.361059656098));
#21931=CARTESIAN_POINT('Ctrl Pts',(271.181638548661,159.955159945194,245.972232660372));
#21932=CARTESIAN_POINT('Ctrl Pts',(271.183113076211,159.95458729014,245.171288638899));
#21933=CARTESIAN_POINT('Ctrl Pts',(271.377233932998,159.86787417663,244.784991571802));
#21934=CARTESIAN_POINT('Ctrl Pts',(272.013257787885,159.697526747734,244.23605360463));
#21935=CARTESIAN_POINT('Ctrl Pts',(272.45983196194,159.632160208303,244.06925769463));
#21936=CARTESIAN_POINT('Ctrl Pts',(272.919178153013,159.656406407913,244.070014088572));
#21937=CARTESIAN_POINT('',(272.893595756463,160.159336843574,246.573593133381));
#21938=CARTESIAN_POINT('',(272.893595838066,160.159335207205,244.573593133703));
#21939=CARTESIAN_POINT('Ctrl Pts',(272.89359575648,160.159336843253,246.573593133703));
#21940=CARTESIAN_POINT('Ctrl Pts',(272.84861813654,160.156998423751,246.573593133777));
#21941=CARTESIAN_POINT('Ctrl Pts',(272.803777913346,160.156762969772,246.570551147));
#21942=CARTESIAN_POINT('Ctrl Pts',(272.715012383882,160.160063357393,246.558577698866));
#21943=CARTESIAN_POINT('Ctrl Pts',(272.671223817618,160.16358947227,246.549670593028));
#21944=CARTESIAN_POINT('Ctrl Pts',(272.54162313439,160.179134800402,246.514389597396));
#21945=CARTESIAN_POINT('Ctrl Pts',(272.459292925889,160.196044952057,246.47971112174));
#21946=CARTESIAN_POINT('Ctrl Pts',(272.331884596952,160.231139310487,246.405940491082));
#21947=CARTESIAN_POINT('Ctrl Pts',(272.283580104659,160.247054870222,246.372086195779));
#21948=CARTESIAN_POINT('Ctrl Pts',(272.212830121178,160.273690718174,246.313003139576));
#21949=CARTESIAN_POINT('Ctrl Pts',(272.188116124322,160.283827212976,246.290206730023));
#21950=CARTESIAN_POINT('Ctrl Pts',(272.141019691395,160.304086208312,246.242334167609));
#21951=CARTESIAN_POINT('Ctrl Pts',(272.118425274288,160.314223541269,246.216956137048));
#21952=CARTESIAN_POINT('Ctrl Pts',(272.057113716637,160.342801676355,246.140681005568));
#21953=CARTESIAN_POINT('Ctrl Pts',(272.021679560313,160.360726146822,246.086958711194));
#21954=CARTESIAN_POINT('Ctrl Pts',(271.96416665625,160.391729751442,245.978032102337));
#21955=CARTESIAN_POINT('Ctrl Pts',(271.941189971409,160.405090586035,245.923416774258));
#21956=CARTESIAN_POINT('Ctrl Pts',(271.893378613539,160.43433731398,245.772513348258));
#21957=CARTESIAN_POINT('Ctrl Pts',(271.877672652427,160.445890623876,245.673483077983));
#21958=CARTESIAN_POINT('Ctrl Pts',(271.877787775074,160.445750590394,245.473008288347));
#21959=CARTESIAN_POINT('Ctrl Pts',(271.893469585958,160.434311803733,245.374193081088));
#21960=CARTESIAN_POINT('Ctrl Pts',(271.941368526616,160.405077356024,245.223303692942));
#21961=CARTESIAN_POINT('Ctrl Pts',(271.964343198474,160.391727578948,245.168765169821));
#21962=CARTESIAN_POINT('Ctrl Pts',(272.021861156968,160.36070465498,245.059926304005));
#21963=CARTESIAN_POINT('Ctrl Pts',(272.057309400142,160.342745164453,245.006226072545));
#21964=CARTESIAN_POINT('Ctrl Pts',(272.118660575559,160.314122358304,244.929954836604));
#21965=CARTESIAN_POINT('Ctrl Pts',(272.141286933469,160.303965616176,244.904560232997));
#21966=CARTESIAN_POINT('Ctrl Pts',(272.188411027287,160.283707825989,244.856699719665));
#21967=CARTESIAN_POINT('Ctrl Pts',(272.213087436914,160.273595046995,244.833955999993));
#21968=CARTESIAN_POINT('Ctrl Pts',(272.283776953734,160.246980411639,244.774957037283));
#21969=CARTESIAN_POINT('Ctrl Pts',(272.332054369033,160.23106401385,244.741137633888));
#21970=CARTESIAN_POINT('Ctrl Pts',(272.459465282786,160.195958053628,244.667392469805));
#21971=CARTESIAN_POINT('Ctrl Pts',(272.541825403793,160.179055115833,244.632719291294));
#21972=CARTESIAN_POINT('Ctrl Pts',(272.67145705261,160.16354874035,244.597463836825));
#21973=CARTESIAN_POINT('Ctrl Pts',(272.715232192116,160.160039330037,244.588569745954));
#21974=CARTESIAN_POINT('Ctrl Pts',(272.803922751181,160.156765637209,244.576624852807));
#21975=CARTESIAN_POINT('Ctrl Pts',(272.848689914664,160.157006237089,244.573593133703));
#21976=CARTESIAN_POINT('Ctrl Pts',(272.893595838066,160.159335207205,244.573593133703));
#21977=CARTESIAN_POINT('',(272.918996157899,159.659984078124,247.073589514835));
#21978=CARTESIAN_POINT('',(272.893595648979,160.159338953007,246.573591021215));
#21979=CARTESIAN_POINT('',(272.918996332872,159.659980853205,244.073593137428));
#21980=CARTESIAN_POINT('Ctrl Pts',(272.918996332834,159.659980853954,244.073593133703));
#21981=CARTESIAN_POINT('Ctrl Pts',(272.684677113858,159.648061814786,244.073325863255));
#21982=CARTESIAN_POINT('Ctrl Pts',(272.464124179613,159.657462336297,244.109847139091));
#21983=CARTESIAN_POINT('Ctrl Pts',(272.158086920106,159.692555569418,244.219811905837));
#21984=CARTESIAN_POINT('Ctrl Pts',(272.060168313579,159.70775995013,244.265663970251));
#21985=CARTESIAN_POINT('Ctrl Pts',(271.872812989298,159.743488842164,244.37576238341));
#21986=CARTESIAN_POINT('Ctrl Pts',(271.784976843385,159.763591097843,244.438626167558));
#21987=CARTESIAN_POINT('Ctrl Pts',(271.524682254253,159.832061411953,244.663127176969));
#21988=CARTESIAN_POINT('Ctrl Pts',(271.397541667612,159.877211097541,244.826245103114));
#21989=CARTESIAN_POINT('Ctrl Pts',(271.229134999604,159.940259016219,245.17938212848));
#21990=CARTESIAN_POINT('Ctrl Pts',(271.187673154397,159.958215997785,245.369501892319));
#21991=CARTESIAN_POINT('Ctrl Pts',(271.186957902735,159.958511753159,245.776239362339));
#21992=CARTESIAN_POINT('Ctrl Pts',(271.228127696939,159.940658438962,245.966395214971));
#21993=CARTESIAN_POINT('Ctrl Pts',(271.354646900259,159.893259013043,246.231809670352));
#21994=CARTESIAN_POINT('Ctrl Pts',(271.407668107912,159.87415637492,246.316977934885));
#21995=CARTESIAN_POINT('Ctrl Pts',(271.504112506007,159.842601973052,246.439775500791));
#21996=CARTESIAN_POINT('Ctrl Pts',(271.539080824339,159.831609459822,246.479882217612));
#21997=CARTESIAN_POINT('Ctrl Pts',(271.614770265428,159.809128983085,246.558444040955));
#21998=CARTESIAN_POINT('Ctrl Pts',(271.656587198068,159.797353514779,246.597842459808));
#21999=CARTESIAN_POINT('Ctrl Pts',(272.039253889,159.696787821332,246.927734975046));
#22000=CARTESIAN_POINT('Ctrl Pts',(272.44884461053,159.636065800518,247.074098313406));
#22001=CARTESIAN_POINT('Ctrl Pts',(272.918996199032,159.659983271947,247.073589666413));
#22002=CARTESIAN_POINT('',(272.893595838066,160.159335207205,244.573593133703));
#22003=CARTESIAN_POINT('Ctrl Pts',(272.537990049465,167.150273777714,244.573616253716));
#22004=CARTESIAN_POINT('Ctrl Pts',(272.270838062775,167.13591464661,244.574119305608));
#22005=CARTESIAN_POINT('Ctrl Pts',(272.017726904027,167.047492757115,244.684408642187));
#22006=CARTESIAN_POINT('Ctrl Pts',(271.661746064792,166.851992276134,245.049508832668));
#22007=CARTESIAN_POINT('Ctrl Pts',(271.556108095729,166.761909243715,245.3079542367));
#22008=CARTESIAN_POINT('Ctrl Pts',(271.556833868663,166.762471981263,245.840603181627));
#22009=CARTESIAN_POINT('Ctrl Pts',(271.662035551128,166.852213542768,246.097805937303));
#22010=CARTESIAN_POINT('Ctrl Pts',(272.018208621965,167.047688871632,246.463441120033));
#22011=CARTESIAN_POINT('Ctrl Pts',(272.272038173957,167.136252218062,246.5735069616));
#22012=CARTESIAN_POINT('Ctrl Pts',(272.806924217017,167.164445601671,246.573630836524));
#22013=CARTESIAN_POINT('Ctrl Pts',(273.066695983064,167.100703248862,246.462788131368));
#22014=CARTESIAN_POINT('Ctrl Pts',(273.439644774456,166.942404373256,246.097309136337));
#22015=CARTESIAN_POINT('Ctrl Pts',(273.55425519788,166.863528512065,245.838717275493));
#22016=CARTESIAN_POINT('Ctrl Pts',(273.553388016837,166.864050599837,245.306031552117));
#22017=CARTESIAN_POINT('Ctrl Pts',(273.439057224836,166.942672865528,245.049122246731));
#22018=CARTESIAN_POINT('Ctrl Pts',(273.066149490319,167.10090686242,244.68404329363));
#22019=CARTESIAN_POINT('Ctrl Pts',(272.805142036156,167.164632908818,244.573113201823));
#22020=CARTESIAN_POINT('Ctrl Pts',(272.537990049465,167.150273777714,244.573616253716));
#22021=CARTESIAN_POINT('Ctrl Pts',(272.512403161391,167.65329248121,244.069947188143));
#22022=CARTESIAN_POINT('Ctrl Pts',(272.053031438508,167.629044968165,244.07070361574));
#22023=CARTESIAN_POINT('Ctrl Pts',(271.615555387453,167.520373390882,244.236543467048));
#22024=CARTESIAN_POINT('Ctrl Pts',(270.998247103352,167.286052004531,244.785537777997));
#22025=CARTESIAN_POINT('Ctrl Pts',(270.814123357274,167.179786452026,245.174161966009));
#22026=CARTESIAN_POINT('Ctrl Pts',(270.815386702198,167.180452195518,245.975086074588));
#22027=CARTESIAN_POINT('Ctrl Pts',(270.998750983871,167.2863139197,246.361841771234));
#22028=CARTESIAN_POINT('Ctrl Pts',(271.616388676161,167.520612064187,246.911640429713));
#22029=CARTESIAN_POINT('Ctrl Pts',(272.05510178248,167.629466589457,247.077144255326));
#22030=CARTESIAN_POINT('Ctrl Pts',(272.974832701618,167.677377583998,247.07733055111));
#22031=CARTESIAN_POINT('Ctrl Pts',(273.419306690832,167.611955975499,246.910658590737));
#22032=CARTESIAN_POINT('Ctrl Pts',(274.055434107672,167.44153383431,246.361094693722));
#22033=CARTESIAN_POINT('Ctrl Pts',(274.250038582589,167.354537348704,245.972250397064));
#22034=CARTESIAN_POINT('Ctrl Pts',(274.248563974356,167.355110010476,245.171270739137));
#22035=CARTESIAN_POINT('Ctrl Pts',(274.054432517953,167.441824198804,244.784956483677));
#22036=CARTESIAN_POINT('Ctrl Pts',(273.418373709719,167.612173236895,244.235994091974));
#22037=CARTESIAN_POINT('Ctrl Pts',(272.971774884274,167.677539994255,244.069190760545));
#22038=CARTESIAN_POINT('Ctrl Pts',(272.512403161391,167.65329248121,244.069947188143));
#22039=CARTESIAN_POINT('',(272.53798895654,167.150295231503,246.573593133381));
#22040=CARTESIAN_POINT('',(272.537988874946,167.150296867873,244.573593133703));
#22041=CARTESIAN_POINT('Ctrl Pts',(272.537988956523,167.150295231825,246.573593133703));
#22042=CARTESIAN_POINT('Ctrl Pts',(272.582966576466,167.152633651326,246.573593133777));
#22043=CARTESIAN_POINT('Ctrl Pts',(272.627806799662,167.152869105306,246.570551147));
#22044=CARTESIAN_POINT('Ctrl Pts',(272.716572329129,167.149568717685,246.558577698866));
#22045=CARTESIAN_POINT('Ctrl Pts',(272.760360895393,167.146042602808,246.549670593028));
#22046=CARTESIAN_POINT('Ctrl Pts',(272.889961578622,167.130497274676,246.514389597396));
#22047=CARTESIAN_POINT('Ctrl Pts',(272.972291787123,167.113587123021,246.47971112174));
#22048=CARTESIAN_POINT('Ctrl Pts',(273.09970011606,167.078492764591,246.405940491082));
#22049=CARTESIAN_POINT('Ctrl Pts',(273.148004608353,167.062577204855,246.372086195779));
#22050=CARTESIAN_POINT('Ctrl Pts',(273.218754591834,167.035941356904,246.313003139576));
#22051=CARTESIAN_POINT('Ctrl Pts',(273.24346858869,167.025804862102,246.290206730023));
#22052=CARTESIAN_POINT('Ctrl Pts',(273.290565021617,167.005545866766,246.242334167609));
#22053=CARTESIAN_POINT('Ctrl Pts',(273.313159438724,166.995408533809,246.216956137048));
#22054=CARTESIAN_POINT('Ctrl Pts',(273.374470996374,166.966830398723,246.140681005568));
#22055=CARTESIAN_POINT('Ctrl Pts',(273.409905152699,166.948905928256,246.086958711195));
#22056=CARTESIAN_POINT('Ctrl Pts',(273.467418056762,166.917902323636,245.978032102338));
#22057=CARTESIAN_POINT('Ctrl Pts',(273.490394741603,166.904541489043,245.923416774259));
#22058=CARTESIAN_POINT('Ctrl Pts',(273.538206099473,166.875294761098,245.772513348258));
#22059=CARTESIAN_POINT('Ctrl Pts',(273.553912060585,166.863741451202,245.673483077984));
#22060=CARTESIAN_POINT('Ctrl Pts',(273.553796937938,166.863881484684,245.473008288348));
#22061=CARTESIAN_POINT('Ctrl Pts',(273.538115127054,166.875320271345,245.374193081089));
#22062=CARTESIAN_POINT('Ctrl Pts',(273.490216186397,166.904554719054,245.223303692942));
#22063=CARTESIAN_POINT('Ctrl Pts',(273.467241514539,166.91790449613,245.168765169821));
#22064=CARTESIAN_POINT('Ctrl Pts',(273.409723556044,166.948927420098,245.059926304005));
#22065=CARTESIAN_POINT('Ctrl Pts',(273.37427531287,166.966886910625,245.006226072545));
#22066=CARTESIAN_POINT('Ctrl Pts',(273.312924137453,166.995509716774,244.929954836604));
#22067=CARTESIAN_POINT('Ctrl Pts',(273.290297779544,167.005666458902,244.904560232997));
#22068=CARTESIAN_POINT('Ctrl Pts',(273.243173685724,167.02592424909,244.856699719664));
#22069=CARTESIAN_POINT('Ctrl Pts',(273.218497276097,167.036037028083,244.833955999992));
#22070=CARTESIAN_POINT('Ctrl Pts',(273.147807759279,167.062651663438,244.774957037284));
#22071=CARTESIAN_POINT('Ctrl Pts',(273.099530343979,167.078568061228,244.741137633888));
#22072=CARTESIAN_POINT('Ctrl Pts',(272.972119430226,167.11367402145,244.667392469805));
#22073=CARTESIAN_POINT('Ctrl Pts',(272.889759309219,167.130576959245,244.632719291294));
#22074=CARTESIAN_POINT('Ctrl Pts',(272.760127660401,167.146083334728,244.597463836825));
#22075=CARTESIAN_POINT('Ctrl Pts',(272.716352520896,167.149592745041,244.588569745954));
#22076=CARTESIAN_POINT('Ctrl Pts',(272.627661961831,167.152866437869,244.576624852807));
#22077=CARTESIAN_POINT('Ctrl Pts',(272.582894798349,167.152625837989,244.573593133703));
#22078=CARTESIAN_POINT('Ctrl Pts',(272.537988874946,167.150296867873,244.573593133703));
#22079=CARTESIAN_POINT('',(272.512586339276,167.649647881398,247.073589202258));
#22080=CARTESIAN_POINT('',(272.537989064033,167.150293122071,246.573591021215));
#22081=CARTESIAN_POINT('',(272.51258838014,167.649651221873,244.073593137428));
#22082=CARTESIAN_POINT('Ctrl Pts',(272.512588380178,167.649651221123,244.073593133703));
#22083=CARTESIAN_POINT('Ctrl Pts',(272.746773917338,167.661563460343,244.073207336743));
#22084=CARTESIAN_POINT('Ctrl Pts',(272.967263075997,167.652182489951,244.109671982816));
#22085=CARTESIAN_POINT('Ctrl Pts',(273.273311423625,167.617102815298,244.219644650044));
#22086=CARTESIAN_POINT('Ctrl Pts',(273.371251311414,167.6019004664,244.26551482214));
#22087=CARTESIAN_POINT('Ctrl Pts',(273.558682837338,167.566163320439,244.375680399037));
#22088=CARTESIAN_POINT('Ctrl Pts',(273.646645002999,167.546032094573,244.438654405421));
#22089=CARTESIAN_POINT('Ctrl Pts',(273.906938958271,167.477559290898,244.663166238249));
#22090=CARTESIAN_POINT('Ctrl Pts',(274.034076078324,167.432409299256,244.826292334005));
#22091=CARTESIAN_POINT('Ctrl Pts',(274.202470426655,167.369364615484,245.179447606592));
#22092=CARTESIAN_POINT('Ctrl Pts',(274.243923553764,167.351411117335,245.369584971744));
#22093=CARTESIAN_POINT('Ctrl Pts',(274.244615114457,167.351125158105,245.776329368437));
#22094=CARTESIAN_POINT('Ctrl Pts',(274.203430535256,167.368984709093,245.966487747264));
#22095=CARTESIAN_POINT('Ctrl Pts',(274.076883746714,167.416392740919,246.231904586228));
#22096=CARTESIAN_POINT('Ctrl Pts',(274.023852437588,167.43549810258,246.317073411003));
#22097=CARTESIAN_POINT('Ctrl Pts',(273.927391417782,167.467055829036,246.439871465846));
#22098=CARTESIAN_POINT('Ctrl Pts',(273.892417314405,167.478049322204,246.479978287074));
#22099=CARTESIAN_POINT('Ctrl Pts',(273.816715804945,167.500531393776,246.55854020209));
#22100=CARTESIAN_POINT('Ctrl Pts',(273.774892281931,167.512307489834,246.597938651966));
#22101=CARTESIAN_POINT('Ctrl Pts',(273.39219560437,167.612869582687,246.927807707392));
#22102=CARTESIAN_POINT('Ctrl Pts',(272.983080973498,167.673583875118,247.074228761836));
#22103=CARTESIAN_POINT('Ctrl Pts',(272.512586298077,167.649648688282,247.073589199254));
#22104=CARTESIAN_POINT('',(272.537988874946,167.150296867873,244.573593133703));
#22105=CARTESIAN_POINT('Origin',(272.918996332834,159.659980853954,245.573593133703));
#22106=CARTESIAN_POINT('Ctrl Pts',(272.893595838066,160.159335207205,244.573593133703));
#22107=CARTESIAN_POINT('Ctrl Pts',(272.994616473054,160.164574472366,244.573593133703));
#22108=CARTESIAN_POINT('Ctrl Pts',(273.093662374227,160.180056064334,244.588926668372));
#22109=CARTESIAN_POINT('Ctrl Pts',(273.219128553104,160.210726797024,244.628234491494));
#22110=CARTESIAN_POINT('Ctrl Pts',(273.249831367943,160.219204367691,244.639604524938));
#22111=CARTESIAN_POINT('Ctrl Pts',(273.407689912623,160.26748834392,244.707242077007));
#22112=CARTESIAN_POINT('Ctrl Pts',(273.51238388592,160.315968713744,244.784746950619));
#22113=CARTESIAN_POINT('Ctrl Pts',(273.605317555611,160.367292821967,244.880838247272));
#22114=CARTESIAN_POINT('Ctrl Pts',(273.616512492842,160.373584974036,244.89301514354));
#22115=CARTESIAN_POINT('Ctrl Pts',(273.638351446563,160.386067565299,244.918011816566));
#22116=CARTESIAN_POINT('Ctrl Pts',(273.648992741935,160.392257403739,244.930834103936));
#22117=CARTESIAN_POINT('Ctrl Pts',(273.698212284866,160.421369893916,244.993308664964));
#22118=CARTESIAN_POINT('Ctrl Pts',(273.732636125182,160.443230582208,245.046721221241));
#22119=CARTESIAN_POINT('Ctrl Pts',(273.788644179573,160.480856811058,245.155343526424));
#22120=CARTESIAN_POINT('Ctrl Pts',(273.811078606603,160.496980228528,245.209956194151));
#22121=CARTESIAN_POINT('Ctrl Pts',(273.844618130314,160.522223407935,245.317836348554));
#22122=CARTESIAN_POINT('Ctrl Pts',(273.856602086653,160.531853954495,245.37057049282));
#22123=CARTESIAN_POINT('Ctrl Pts',(273.871541519234,160.544235433038,245.473637636457));
#22124=CARTESIAN_POINT('Ctrl Pts',(273.875146524561,160.547467285949,245.523509871061));
#22125=CARTESIAN_POINT('Ctrl Pts',(273.875152125532,160.547339455183,245.66744290748));
#22126=CARTESIAN_POINT('Ctrl Pts',(273.862589234204,160.535782206681,245.766443228677));
#22127=CARTESIAN_POINT('Ctrl Pts',(273.816003541422,160.500425343,245.923804651633));
#22128=CARTESIAN_POINT('Ctrl Pts',(273.794496765221,160.48482593628,245.978365805299));
#22129=CARTESIAN_POINT('Ctrl Pts',(273.74041500634,160.448146636058,246.087229534119));
#22130=CARTESIAN_POINT('Ctrl Pts',(273.706974062563,160.426691435871,246.14092965317));
#22131=CARTESIAN_POINT('Ctrl Pts',(273.648845164208,160.391985299248,246.21720597302));
#22132=CARTESIAN_POINT('Ctrl Pts',(273.627363573115,160.379578351121,246.242605470456));
#22133=CARTESIAN_POINT('Ctrl Pts',(273.582546114185,160.354632982326,246.290460601382));
#22134=CARTESIAN_POINT('Ctrl Pts',(273.55901778022,160.342061412841,246.313212577002));
#22135=CARTESIAN_POINT('Ctrl Pts',(273.491409518233,160.308447258061,246.372197845411));
#22136=CARTESIAN_POINT('Ctrl Pts',(273.445024697867,160.287769251785,246.406000105603));
#22137=CARTESIAN_POINT('Ctrl Pts',(273.358606430672,160.254271830567,246.457744032174));
#22138=CARTESIAN_POINT('Ctrl Pts',(273.319995253228,160.240805734068,246.477508148981));
#22139=CARTESIAN_POINT('Ctrl Pts',(273.249957547624,160.219355296728,246.507530839586));
#22140=CARTESIAN_POINT('Ctrl Pts',(273.219244688596,160.210860905962,246.518909668632));
#22141=CARTESIAN_POINT('Ctrl Pts',(273.093736058858,160.180122398011,246.558247879177));
#22142=CARTESIAN_POINT('Ctrl Pts',(272.994663057878,160.164591406496,246.573593133538));
#22143=CARTESIAN_POINT('Ctrl Pts',(272.89359575648,160.159336843253,246.573593133703));
#22144=CARTESIAN_POINT('',(272.918996332834,159.659980853954,246.573593133703));
#22145=CARTESIAN_POINT('Ctrl Pts',(272.537988874946,167.150296867873,244.573593133703));
#22146=CARTESIAN_POINT('Ctrl Pts',(272.436968239958,167.145057602712,244.573593133703));
#22147=CARTESIAN_POINT('Ctrl Pts',(272.337922338785,167.129576010743,244.588926668372));
#22148=CARTESIAN_POINT('Ctrl Pts',(272.212456159909,167.098905278054,244.628234491494));
#22149=CARTESIAN_POINT('Ctrl Pts',(272.18175334507,167.090427707387,244.639604524937));
#22150=CARTESIAN_POINT('Ctrl Pts',(272.023894800388,167.042143731157,244.707242077008));
#22151=CARTESIAN_POINT('Ctrl Pts',(271.919200827091,166.993663361333,244.78474695062));
#22152=CARTESIAN_POINT('Ctrl Pts',(271.826267157402,166.942339253112,244.880838247271));
#22153=CARTESIAN_POINT('Ctrl Pts',(271.81507222017,166.936047101043,244.893015143539));
#22154=CARTESIAN_POINT('Ctrl Pts',(271.793233266447,166.923564509778,244.918011816568));
#22155=CARTESIAN_POINT('Ctrl Pts',(271.782591971076,166.917374671339,244.930834103937));
#22156=CARTESIAN_POINT('Ctrl Pts',(271.733372428147,166.888262181162,244.993308664963));
#22157=CARTESIAN_POINT('Ctrl Pts',(271.69894858783,166.86640149287,245.046721221241));
#22158=CARTESIAN_POINT('Ctrl Pts',(271.642940533439,166.82877526402,245.155343526424));
#22159=CARTESIAN_POINT('Ctrl Pts',(271.620506106409,166.81265184655,245.209956194151));
#22160=CARTESIAN_POINT('Ctrl Pts',(271.586966582698,166.787408667143,245.317836348554));
#22161=CARTESIAN_POINT('Ctrl Pts',(271.574982626359,166.777778120583,245.37057049282));
#22162=CARTESIAN_POINT('Ctrl Pts',(271.560043193778,166.76539664204,245.473637636457));
#22163=CARTESIAN_POINT('Ctrl Pts',(271.556438188452,166.762164789129,245.523509871061));
#22164=CARTESIAN_POINT('Ctrl Pts',(271.55643258748,166.762292619895,245.667442907478));
#22165=CARTESIAN_POINT('Ctrl Pts',(271.568995478808,166.773849868396,245.766443228675));
#22166=CARTESIAN_POINT('Ctrl Pts',(271.61558117159,166.809206732078,245.923804651634));
#22167=CARTESIAN_POINT('Ctrl Pts',(271.637087947791,166.824806138798,245.978365805299));
#22168=CARTESIAN_POINT('Ctrl Pts',(271.691169706672,166.86148543902,246.087229534119));
#22169=CARTESIAN_POINT('Ctrl Pts',(271.724610650449,166.882940639207,246.140929653169));
#22170=CARTESIAN_POINT('Ctrl Pts',(271.782739548805,166.91764677583,246.21720597302));
#22171=CARTESIAN_POINT('Ctrl Pts',(271.804221139898,166.930053723957,246.242605470457));
#22172=CARTESIAN_POINT('Ctrl Pts',(271.849038598827,166.954999092752,246.290460601381));
#22173=CARTESIAN_POINT('Ctrl Pts',(271.872566932792,166.967570662237,246.313212577002));
#22174=CARTESIAN_POINT('Ctrl Pts',(271.940175194779,167.001184817018,246.372197845412));
#22175=CARTESIAN_POINT('Ctrl Pts',(271.986560015145,167.021862823293,246.406000105603));
#22176=CARTESIAN_POINT('Ctrl Pts',(272.07297828234,167.05536024451,246.457744032173));
#22177=CARTESIAN_POINT('Ctrl Pts',(272.111589459784,167.06882634101,246.477508148981));
#22178=CARTESIAN_POINT('Ctrl Pts',(272.181627165386,167.09027677835,246.507530839585));
#22179=CARTESIAN_POINT('Ctrl Pts',(272.212340024415,167.098771169116,246.518909668632));
#22180=CARTESIAN_POINT('Ctrl Pts',(272.337848654154,167.129509677067,246.558247879178));
#22181=CARTESIAN_POINT('Ctrl Pts',(272.436921655125,167.145040668581,246.573593133537));
#22182=CARTESIAN_POINT('Ctrl Pts',(272.537988956524,167.150295231825,246.573593133703));
#22183=CARTESIAN_POINT('Origin',(272.715792356506,163.654816037539,244.073593133703));
#22184=CARTESIAN_POINT('Origin',(272.715792356506,163.654816037539,244.073593133703));
#22185=CARTESIAN_POINT('',(272.860336397617,160.81319043826,242.073593133703));
#22186=CARTESIAN_POINT('',(272.918996332834,159.659980853954,244.073593133703));
#22187=CARTESIAN_POINT('Origin',(272.715792356506,163.654816037539,242.073593133703));
#22188=CARTESIAN_POINT('Origin',(272.715792356506,163.654816037539,244.073593133703));
#22189=CARTESIAN_POINT('Origin',(272.715792356506,163.654816037539,275.073593133703));
#22190=CARTESIAN_POINT('',(272.918996332834,159.659980853954,271.473593133703));
#22191=CARTESIAN_POINT('Origin',(272.715792356506,163.654816037539,271.473593133703));
#22192=CARTESIAN_POINT('',(272.918996332834,159.659980853954,275.073593133703));
#22193=CARTESIAN_POINT('Ctrl Pts',(272.918996199032,159.659983271947,247.073589666413));
#22194=CARTESIAN_POINT('Ctrl Pts',(273.153859212278,159.671927547002,247.073336255209));
#22195=CARTESIAN_POINT('Ctrl Pts',(273.372660288957,159.70377047134,247.036490765957));
#22196=CARTESIAN_POINT('Ctrl Pts',(273.673764602282,159.769864517502,246.926335097092));
#22197=CARTESIAN_POINT('Ctrl Pts',(273.769654298301,159.794962976943,246.880468634973));
#22198=CARTESIAN_POINT('Ctrl Pts',(273.952361524276,159.849558183586,246.770439899072));
#22199=CARTESIAN_POINT('Ctrl Pts',(274.037664357212,159.878484631533,246.707630692229));
#22200=CARTESIAN_POINT('Ctrl Pts',(274.28926051078,159.972928496558,246.48357204053));
#22201=CARTESIAN_POINT('Ctrl Pts',(274.410961576191,160.030666872069,246.320599865048));
#22202=CARTESIAN_POINT('Ctrl Pts',(274.571815296306,160.110350675333,245.967456032054));
#22203=CARTESIAN_POINT('Ctrl Pts',(274.611156238513,160.132374288436,245.777012017024));
#22204=CARTESIAN_POINT('Ctrl Pts',(274.611768955062,160.132704049148,245.370016379345));
#22205=CARTESIAN_POINT('Ctrl Pts',(274.572653255307,160.110784343642,245.179908713947));
#22206=CARTESIAN_POINT('Ctrl Pts',(274.451745863215,160.050861447959,244.914832446015));
#22207=CARTESIAN_POINT('Ctrl Pts',(274.401003972674,160.026507080061,244.829821228398));
#22208=CARTESIAN_POINT('Ctrl Pts',(274.308388844366,159.98537773619,244.707325709514));
#22209=CARTESIAN_POINT('Ctrl Pts',(274.274764428741,159.970910463762,244.667330754476));
#22210=CARTESIAN_POINT('Ctrl Pts',(274.201852739805,159.940899138132,244.58901461358));
#22211=CARTESIAN_POINT('Ctrl Pts',(274.161544916096,159.924972533663,244.549787659307));
#22212=CARTESIAN_POINT('Ctrl Pts',(273.791046797412,159.786025320408,244.220670026599));
#22213=CARTESIAN_POINT('Ctrl Pts',(273.387920330164,159.683833457748,244.074128067476));
#22214=CARTESIAN_POINT('Ctrl Pts',(272.918996332834,159.659980853954,244.073593133703));
#22215=CARTESIAN_POINT('Ctrl Pts',(272.512586298077,167.649648688282,247.073589199254));
#22216=CARTESIAN_POINT('Ctrl Pts',(272.277568574454,167.637696415093,247.073269716825));
#22217=CARTESIAN_POINT('Ctrl Pts',(272.058691859226,167.605823019205,247.036390577157));
#22218=CARTESIAN_POINT('Ctrl Pts',(271.757589019498,167.539710588633,246.926232368273));
#22219=CARTESIAN_POINT('Ctrl Pts',(271.661718756569,167.514610376932,246.880373048748));
#22220=CARTESIAN_POINT('Ctrl Pts',(271.524744064579,167.473673830181,246.797874194614));
#22221=CARTESIAN_POINT('Ctrl Pts',(271.480222547247,167.459479498864,246.768089597428));
#22222=CARTESIAN_POINT('Ctrl Pts',(271.393448260767,167.430197197099,246.703950444775));
#22223=CARTESIAN_POINT('Ctrl Pts',(271.352014487236,167.415416685365,246.670325582074));
#22224=CARTESIAN_POINT('Ctrl Pts',(271.142288519241,167.336690915954,246.483479342273));
#22225=CARTESIAN_POINT('Ctrl Pts',(271.020563643374,167.278937434362,246.320448669587));
#22226=CARTESIAN_POINT('Ctrl Pts',(270.859706968011,167.199248759337,245.967279962524));
#22227=CARTESIAN_POINT('Ctrl Pts',(270.820388289757,167.177236159359,245.776985842833));
#22228=CARTESIAN_POINT('Ctrl Pts',(270.819857455755,167.176950467535,245.369914584485));
#22229=CARTESIAN_POINT('Ctrl Pts',(270.858993403178,167.198880150875,245.179793889859));
#22230=CARTESIAN_POINT('Ctrl Pts',(270.979899936523,167.258800041995,244.914735249744));
#22231=CARTESIAN_POINT('Ctrl Pts',(271.03063625638,167.283150543605,244.829736103342));
#22232=CARTESIAN_POINT('Ctrl Pts',(271.123234505968,167.324271049542,244.707267984196));
#22233=CARTESIAN_POINT('Ctrl Pts',(271.156851871753,167.338734878646,244.667283711224));
#22234=CARTESIAN_POINT('Ctrl Pts',(271.22974649002,167.368738646529,244.588992032097));
#22235=CARTESIAN_POINT('Ctrl Pts',(271.270071590961,167.38467151604,244.54975425391));
#22236=CARTESIAN_POINT('Ctrl Pts',(271.640320174432,167.523524687871,244.220906926231));
#22237=CARTESIAN_POINT('Ctrl Pts',(272.043430543987,167.625786722725,244.074366090943));
#22238=CARTESIAN_POINT('Ctrl Pts',(272.512588380178,167.649651221123,244.073593133703));
#22239=CARTESIAN_POINT('Origin',(272.715792356506,163.654816037539,271.473593133703));
#22240=CARTESIAN_POINT('',(272.949476929283,159.060755576417,272.073593133703));
#22241=CARTESIAN_POINT('Origin',(272.715792356506,163.654816037539,272.073593133703));
#22242=CARTESIAN_POINT('Origin',(272.949476929283,159.060755576417,271.473593133703));
#22243=CARTESIAN_POINT('Origin',(272.715792356506,163.654816037539,275.073593133703));
#22244=CARTESIAN_POINT('',(272.360185397933,170.645777608812,274.073593133703));
#22245=CARTESIAN_POINT('',(273.071399315079,156.663854466266,274.073593133703));
#22246=CARTESIAN_POINT('Origin',(272.715792356506,163.654816037539,274.073593133703));
#22247=CARTESIAN_POINT('Origin',(272.715792356506,163.654816037539,274.073593133703));
#22248=CARTESIAN_POINT('',(273.071399315079,156.663854466266,272.073593133703));
#22249=CARTESIAN_POINT('',(273.071399315079,156.663854466266,275.073593133703));
#22250=CARTESIAN_POINT('Origin',(272.715792356506,163.654816037539,272.073593133703));
#22251=CARTESIAN_POINT('Origin',(272.715792356506,163.654816037539,275.073593133703));
#22252=CARTESIAN_POINT('',(272.410986392015,169.647068812916,275.073593133703));
#22253=CARTESIAN_POINT('',(272.410986392015,169.647068812916,275.073593133703));
#22254=CARTESIAN_POINT('Origin',(272.715792356506,163.654816037539,275.073593133703));
#22255=CARTESIAN_POINT('Origin',(272.715792356506,163.654816037539,275.073593133703));
#22256=CARTESIAN_POINT('Origin',(265.724830785233,163.299209078966,272.073593133703));
#22257=CARTESIAN_POINT('Origin',(269.874166757227,163.510271996428,242.073593133703));
#22258=CARTESIAN_POINT('Ctrl Pts',(272.537990127326,167.15027224704,244.573617786368));
#22259=CARTESIAN_POINT('Ctrl Pts',(272.270838725555,167.135913146026,244.57412083749));
#22260=CARTESIAN_POINT('Ctrl Pts',(272.017728127825,167.04749131815,244.68441000503));
#22261=CARTESIAN_POINT('Ctrl Pts',(271.661748083804,166.851990955301,245.049509635926));
#22262=CARTESIAN_POINT('Ctrl Pts',(271.55611035357,166.761907972125,245.307954643826));
#22263=CARTESIAN_POINT('Ctrl Pts',(271.556836124868,166.762470709359,245.840602772399));
#22264=CARTESIAN_POINT('Ctrl Pts',(271.662037569487,166.852212221811,246.097805133848));
#22265=CARTESIAN_POINT('Ctrl Pts',(272.018209844694,167.047687432538,246.463439756173));
#22266=CARTESIAN_POINT('Ctrl Pts',(272.272038834089,167.136250717223,246.573505429044));
#22267=CARTESIAN_POINT('Ctrl Pts',(272.806923706075,167.164444040832,246.573629303778));
#22268=CARTESIAN_POINT('Ctrl Pts',(273.066694910078,167.100701693133,246.462786768509));
#22269=CARTESIAN_POINT('Ctrl Pts',(273.439642900624,166.942402854417,246.097308333644));
#22270=CARTESIAN_POINT('Ctrl Pts',(273.554253080628,166.863527017937,245.838716869155));
#22271=CARTESIAN_POINT('Ctrl Pts',(273.553385901434,166.864049105555,245.306031962191));
#22272=CARTESIAN_POINT('Ctrl Pts',(273.439055352264,166.942671346622,245.049123050581));
#22273=CARTESIAN_POINT('Ctrl Pts',(273.06614841851,167.100905306649,244.684044657033));
#22274=CARTESIAN_POINT('Ctrl Pts',(272.805141529096,167.164631348054,244.573114735247));
#22275=CARTESIAN_POINT('Ctrl Pts',(272.537990127326,167.15027224704,244.573617786368));
#22276=CARTESIAN_POINT('Ctrl Pts',(272.512392795351,167.653496269653,244.069743136217));
#22277=CARTESIAN_POINT('Ctrl Pts',(272.052943198304,167.629244750519,244.070499666465));
#22278=CARTESIAN_POINT('Ctrl Pts',(271.615392455326,167.52056496946,244.236362023006));
#22279=CARTESIAN_POINT('Ctrl Pts',(270.99797829939,167.28622785556,244.785430835153));
#22280=CARTESIAN_POINT('Ctrl Pts',(270.813822756294,167.179955747015,245.17410776262));
#22281=CARTESIAN_POINT('Ctrl Pts',(270.815086319005,167.180621532238,245.975140557769));
#22282=CARTESIAN_POINT('Ctrl Pts',(270.998482266767,167.286489787197,246.361948740322));
#22283=CARTESIAN_POINT('Ctrl Pts',(271.616225886466,167.520803660008,246.911822009124));
#22284=CARTESIAN_POINT('Ctrl Pts',(272.055013894835,167.629666405863,247.07734829438));
#22285=CARTESIAN_POINT('Ctrl Pts',(272.974900726542,167.677585388617,247.077534615452));
#22286=CARTESIAN_POINT('Ctrl Pts',(273.419449544341,167.6121630998,246.91084003692));
#22287=CARTESIAN_POINT('Ctrl Pts',(274.055683582988,167.441736047101,246.361201561415));
#22288=CARTESIAN_POINT('Ctrl Pts',(274.25032046597,167.354736271579,245.972304495464));
#22289=CARTESIAN_POINT('Ctrl Pts',(274.24884561165,167.35530895384,245.171216143361));
#22290=CARTESIAN_POINT('Ctrl Pts',(274.054681825528,167.442026420456,244.784849461951));
#22291=CARTESIAN_POINT('Ctrl Pts',(273.418516406651,167.612380366725,244.235812573376));
#22292=CARTESIAN_POINT('Ctrl Pts',(272.971842392397,167.677747788788,244.06898660597));
#22293=CARTESIAN_POINT('Ctrl Pts',(272.512392795351,167.653496269653,244.069743136217));
#22294=CARTESIAN_POINT('Ctrl Pts',(272.893594585687,160.159359828037,244.573617786368));
#22295=CARTESIAN_POINT('Ctrl Pts',(273.160745987457,160.173718929051,244.57412083749));
#22296=CARTESIAN_POINT('Ctrl Pts',(273.413856585187,160.262140756928,244.68441000503));
#22297=CARTESIAN_POINT('Ctrl Pts',(273.769836629208,160.457641119777,245.049509635926));
#22298=CARTESIAN_POINT('Ctrl Pts',(273.875474359442,160.547724102953,245.307954643826));
#22299=CARTESIAN_POINT('Ctrl Pts',(273.874748588144,160.547161365719,245.840602772399));
#22300=CARTESIAN_POINT('Ctrl Pts',(273.769547143525,160.457419853267,246.097805133848));
#22301=CARTESIAN_POINT('Ctrl Pts',(273.413374868318,160.26194464254,246.463439756173));
#22302=CARTESIAN_POINT('Ctrl Pts',(273.159545878923,160.173381357855,246.573505429044));
#22303=CARTESIAN_POINT('Ctrl Pts',(272.624661006937,160.145188034246,246.573629303778));
#22304=CARTESIAN_POINT('Ctrl Pts',(272.364889802934,160.208930381945,246.462786768509));
#22305=CARTESIAN_POINT('Ctrl Pts',(271.991941812388,160.367229220661,246.097308333644));
#22306=CARTESIAN_POINT('Ctrl Pts',(271.877331632384,160.446105057141,245.838716869155));
#22307=CARTESIAN_POINT('Ctrl Pts',(271.878198811578,160.445582969523,245.306031962191));
#22308=CARTESIAN_POINT('Ctrl Pts',(271.992529360748,160.366960728456,245.049123050581));
#22309=CARTESIAN_POINT('Ctrl Pts',(272.365436294502,160.208726768429,244.684044657033));
#22310=CARTESIAN_POINT('Ctrl Pts',(272.626443183916,160.145000727024,244.573114735247));
#22311=CARTESIAN_POINT('Ctrl Pts',(272.893594585687,160.159359828037,244.573617786368));
#22312=CARTESIAN_POINT('Ctrl Pts',(272.919202378768,159.655930148048,244.069537212942));
#22313=CARTESIAN_POINT('Ctrl Pts',(273.378730564158,159.680185710011,244.070293846782));
#22314=CARTESIAN_POINT('Ctrl Pts',(273.816356684055,159.788873770082,244.236178914949));
#22315=CARTESIAN_POINT('Ctrl Pts',(274.433877682772,160.023226755769,244.785322911543));
#22316=CARTESIAN_POINT('Ctrl Pts',(274.618065314493,160.129505480478,245.174053062134));
#22317=CARTESIAN_POINT('Ctrl Pts',(274.616801531998,160.128839653142,245.975195540614));
#22318=CARTESIAN_POINT('Ctrl Pts',(274.433373627741,160.022964807513,246.362056690417));
#22319=CARTESIAN_POINT('Ctrl Pts',(273.815523109177,159.788635062134,246.91200525379));
#22320=CARTESIAN_POINT('Ctrl Pts',(273.376659511836,159.679764020304,247.077554204665));
#22321=CARTESIAN_POINT('Ctrl Pts',(272.456615337694,159.631836976076,247.077740551258));
#22322=CARTESIAN_POINT('Ctrl Pts',(272.011991005059,159.697259951451,246.911023147137));
#22323=CARTESIAN_POINT('Ctrl Pts',(271.375649366784,159.867691960703,246.361309409185));
#22324=CARTESIAN_POINT('Ctrl Pts',(271.180979778523,159.954695056313,245.972359089997));
#22325=CARTESIAN_POINT('Ctrl Pts',(271.182454881187,159.954122353375,245.17116104689));
#22326=CARTESIAN_POINT('Ctrl Pts',(271.376651293522,159.867401578405,244.784741458735));
#22327=CARTESIAN_POINT('Ctrl Pts',(272.012924300764,159.697042678946,244.235629390082));
#22328=CARTESIAN_POINT('Ctrl Pts',(272.459674193378,159.631674586084,244.068780579103));
#22329=CARTESIAN_POINT('Ctrl Pts',(272.919202378768,159.655930148048,244.069537212942));
#27766=UNCERTAINTY_MEASURE_WITH_UNIT(LENGTH_MEASURE(0.01),#27808,
'DISTANCE_ACCURACY_VALUE',
'Maximum model space distance between geometric entities at asserted c
onnectivities');
#27778=UNCERTAINTY_MEASURE_WITH_UNIT(LENGTH_MEASURE(0.01),#27808,
'DISTANCE_ACCURACY_VALUE',
'Maximum model space distance between geometric entities at asserted c
onnectivities');
#27795=(
GEOMETRIC_REPRESENTATION_CONTEXT(3)
GLOBAL_UNCERTAINTY_ASSIGNED_CONTEXT((#27766))
GLOBAL_UNIT_ASSIGNED_CONTEXT((#27808,#27810,#27811))
REPRESENTATION_CONTEXT('','3D')
);
#27807=(
GEOMETRIC_REPRESENTATION_CONTEXT(3)
GLOBAL_UNCERTAINTY_ASSIGNED_CONTEXT((#27778))
GLOBAL_UNIT_ASSIGNED_CONTEXT((#27808,#27810,#27811))
REPRESENTATION_CONTEXT('','3D')
);
#27808=(
LENGTH_UNIT()
NAMED_UNIT(*)
SI_UNIT(.MILLI.,.METRE.)
);
#27810=(
NAMED_UNIT(*)
PLANE_ANGLE_UNIT()
SI_UNIT($,.RADIAN.)
);
#27811=(
NAMED_UNIT(*)
SI_UNIT($,.STERADIAN.)
SOLID_ANGLE_UNIT()
);
#27828=SHAPE_DEFINITION_REPRESENTATION(#27861,#27915);
#27861=PRODUCT_DEFINITION_SHAPE('',$,#27944);
#27915=SHAPE_REPRESENTATION('',(#13263),#27795);
#27927=PRODUCT_DEFINITION_CONTEXT('part definition',#28013,'design');
#27944=PRODUCT_DEFINITION('Pump Pins','Pump Pins',#27972,#27927);
#27972=PRODUCT_DEFINITION_FORMATION('',$,#28031);
#28013=APPLICATION_CONTEXT('Managed model based 3d engineering');
#28014=PRODUCT_CONTEXT('part definition',#28013,'mechanical');
#28031=PRODUCT('Pump Pins','Pump Pins',$,(#28014));
#28057=COLOUR_RGB('Light Blue',0.38,0.62,0.78);
#28058=FILL_AREA_STYLE_COLOUR('',#28057);
#28059=FILL_AREA_STYLE('',(#28058));
#28060=SURFACE_STYLE_FILL_AREA(#28059);
#28061=SURFACE_SIDE_STYLE('',(#28060));
#28062=SURFACE_STYLE_USAGE(.BOTH.,#28061);
#28063=PRESENTATION_STYLE_ASSIGNMENT((#28062));
ENDSEC;
END-ISO-10303-21;
